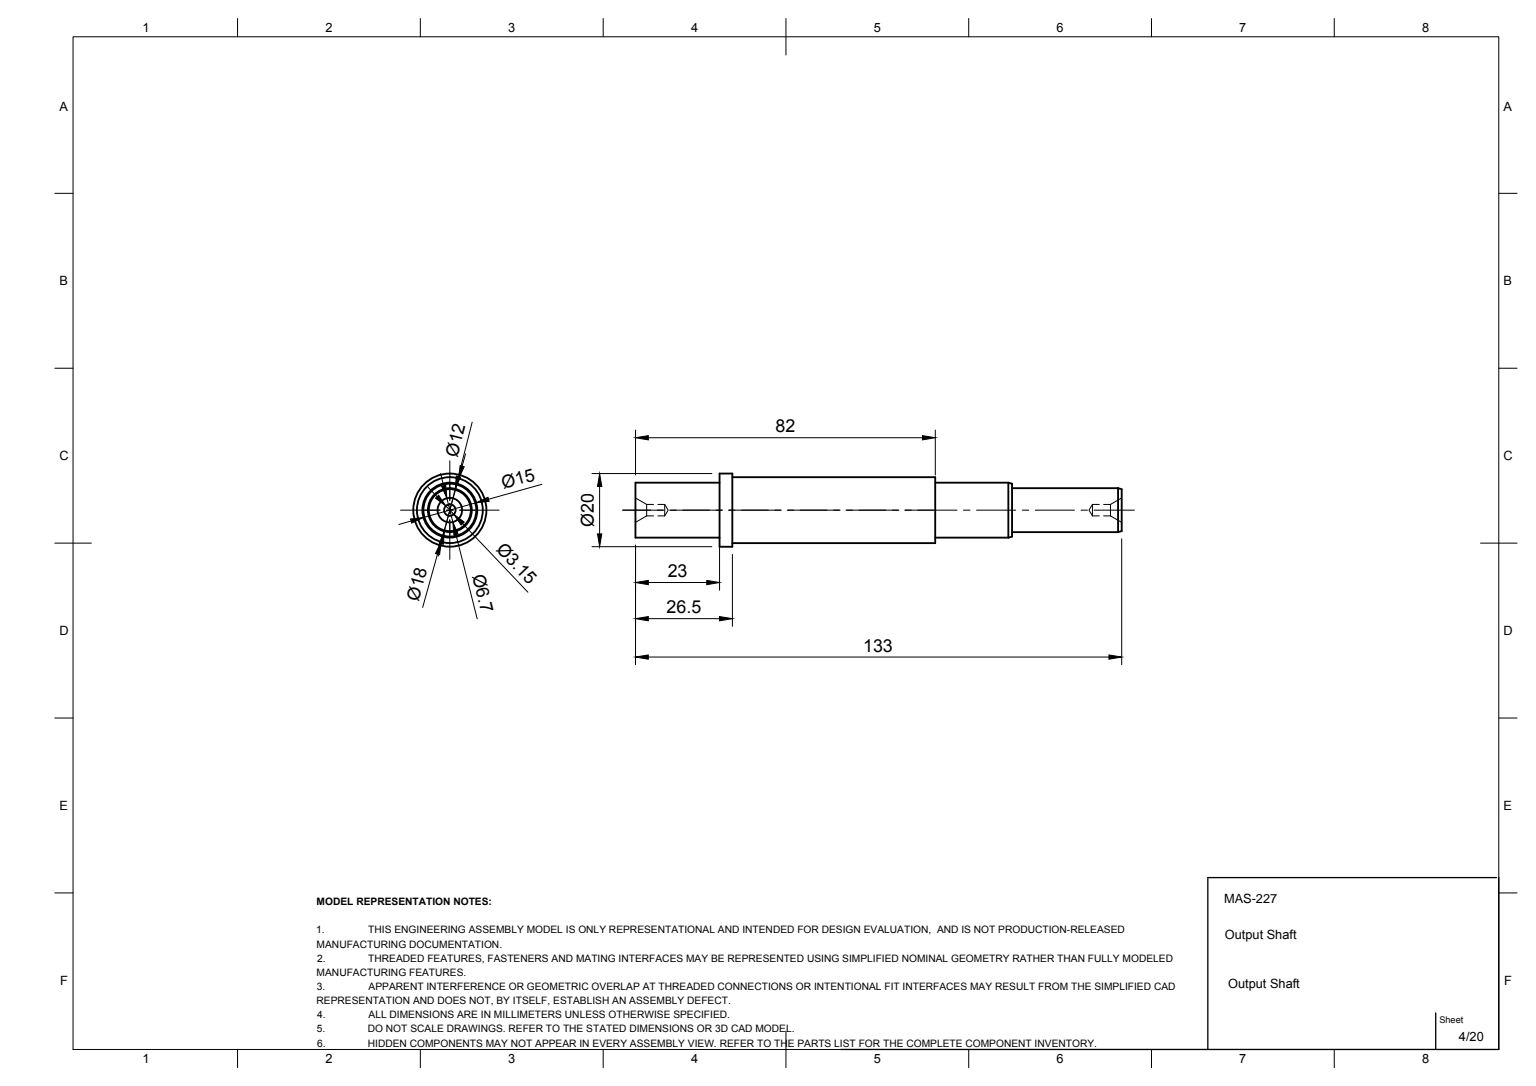
ISO-10303-21;
HEADER;
FILE_DESCRIPTION (('STEP AP214'),
    '1' );
FILE_NAME ( 'Output Shaft.step', '2026-10-06T08:24:41', ( '' ), ( '' ), 'STEP AP214', 'Unspecified', '' );
FILE_SCHEMA (( 'AUTOMOTIVE_DESIGN' ));
ENDSEC;
DATA;
#45=EDGE_CURVE ( 'NONE', #18347, #8484, #23181, .T. ) ;
#57=EDGE_CURVE ( 'NONE', #14897, #14790, #10537, .T. ) ;
#66=DIRECTION ( 'NONE',  ( 0.000000000000000000, 0.000000000000000000, 1.000000000000000000 ) ) ;
#83=DIRECTION ( 'NONE',  ( 0.000000000000000000, 0.000000000000000000, 1.000000000000000000 ) ) ;
#155=CARTESIAN_POINT ( 'NONE',  ( 0.000000000000000000, 0.000000000000000000, 0.9055118110027171596 ) ) ;
#170=CIRCLE ( 'NONE', #27197, 0.2952755905264887182 ) ;
#187=ORIENTED_EDGE ( 'NONE', *, *, #16548, .F. ) ;
#191=ORIENTED_EDGE ( 'NONE', *, *, #12482, .T. ) ;
#231=DIRECTION ( 'NONE',  ( 0.000000000000000000, 0.000000000000000000, 1.000000000000000000 ) ) ;
#281=FACE_OUTER_BOUND ( 'NONE', #3824, .T. ) ;
#333=VERTEX_POINT ( 'NONE', #9774 ) ;
#337=CONICAL_SURFACE ( 'NONE', #25107, 0.06200787401574805319, 1.029744258088332254 ) ;
#346=CARTESIAN_POINT ( 'NONE',  ( 0.06200787401574806013, 0.000000000000000000, 0.7844728274238290666 ) ) ;
#347=ORIENTED_EDGE ( 'NONE', *, *, #11626, .F. ) ;
#395=DIRECTION ( 'NONE',  ( 1.000000000000000000, 0.000000000000000000, 0.000000000000000000 ) ) ;
#427=LINE ( 'NONE', #11141, #5205 ) ;
#455=EDGE_LOOP ( 'NONE', ( #21563, #19160, #191, #7147 ) ) ;
#458=AXIS2_PLACEMENT_3D ( 'NONE', #6185, #12523, #23694 ) ;
#486=DIRECTION ( 'NONE',  ( 1.000000000000000000, 0.000000000000000000, 0.000000000000000000 ) ) ;
#504=LINE ( 'NONE', #11227, #20509 ) ;
#530=CARTESIAN_POINT ( 'NONE',  ( 0.000000000000000000, 0.000000000000000000, -3.110236220451535694 ) ) ;
#576=ORIENTED_EDGE ( 'NONE', *, *, #1922, .T. ) ;
#611=AXIS2_PLACEMENT_3D ( 'NONE', #25131, #20899, #5796 ) ;
#652=CYLINDRICAL_SURFACE ( 'NONE', #15066, 0.2952755905264887182 ) ;
#664=DIRECTION ( 'NONE',  ( 0.000000000000000000, 0.000000000000000000, 1.000000000000000000 ) ) ;
#666=EDGE_CURVE ( 'NONE', #8687, #1454, #4948, .T. ) ;
#667=VECTOR ( 'NONE', #27557, 39.37007874015748143 ) ;
#685=DIRECTION ( 'NONE',  ( 0.000000000000000000, 0.000000000000000000, 1.000000000000000000 ) ) ;
#716=AXIS2_PLACEMENT_3D ( 'NONE', #13335, #23940, #21541 ) ;
#783=VERTEX_POINT ( 'NONE', #2370 ) ;
#786=ORIENTED_EDGE ( 'NONE', *, *, #1340, .T. ) ;
#806=CARTESIAN_POINT ( 'NONE',  ( -0.2952755905264887182, 3.616083068046089993E-17, -4.330708661417323135 ) ) ;
#815=DIRECTION ( 'NONE',  ( 1.000000000000000000, 0.000000000000000000, 0.000000000000000000 ) ) ;
#858=VERTEX_POINT ( 'NONE', #2113 ) ;
#924=DIRECTION ( 'NONE',  ( 1.000000000000000000, 0.000000000000000000, 0.000000000000000000 ) ) ;
#988=DIRECTION ( 'NONE',  ( 1.000000000000000000, 0.000000000000000000, 0.000000000000000000 ) ) ;
#1066=CIRCLE ( 'NONE', #3291, 0.06200787401574806013 ) ;
#1135=CARTESIAN_POINT ( 'NONE',  ( 0.000000000000000000, 0.000000000000000000, -0.1377952755696461029 ) ) ;
#1148=LENGTH_MEASURE_WITH_UNIT ( LENGTH_MEASURE( 0.02539999999999999897 ), #16121 ) ;
#1149=AXIS2_PLACEMENT_3D ( 'NONE', #9958, #18559, #8409 ) ;
#1155=ORIENTED_EDGE ( 'NONE', *, *, #18449, .F. ) ;
#1163=AXIS2_PLACEMENT_3D ( 'NONE', #5767, #10124, #27373 ) ;
#1170=VECTOR ( 'NONE', #19085, 39.37007874015748143 ) ;
#1200=ORIENTED_EDGE ( 'NONE', *, *, #18449, .T. ) ;
#1297=DIRECTION ( 'NONE',  ( 0.000000000000000000, 0.000000000000000000, 1.000000000000000000 ) ) ;
#1299=CARTESIAN_POINT ( 'NONE',  ( 0.3543307086367249448, 0.000000000000000000, -2.322834645648385710 ) ) ;
#1340=EDGE_CURVE ( 'NONE', #2005, #10433, #10148, .T. ) ;
#1368=VECTOR ( 'NONE', #4932, 39.37007874015748143 ) ;
#1388=VERTEX_POINT ( 'NONE', #17057 ) ;
#1454=VERTEX_POINT ( 'NONE', #8971 ) ;
#1460=CARTESIAN_POINT ( 'NONE',  ( -0.2952755905264887182, 3.616083068046089993E-17, -3.110236220451535694 ) ) ;
#1530=ORIENTED_EDGE ( 'NONE', *, *, #9947, .T. ) ;
#1547=DIRECTION ( 'NONE',  ( 0.000000000000000000, 0.000000000000000000, 1.000000000000000000 ) ) ;
#1562=DIRECTION ( 'NONE',  ( 0.000000000000000000, 0.000000000000000000, 1.000000000000000000 ) ) ;
#1604=AXIS2_PLACEMENT_3D ( 'NONE', #9998, #20742, #23148 ) ;
#1728=AXIS2_PLACEMENT_3D ( 'NONE', #26105, #21872, #19190 ) ;
#1815=EDGE_LOOP ( 'NONE', ( #12372, #8684, #25819, #8751 ) ) ;
#1830=ADVANCED_FACE ( 'NONE', ( #7380 ), #27323, .F. ) ;
#1833=LINE ( 'NONE', #12286, #667 ) ;
#1876=EDGE_CURVE ( 'NONE', #10634, #15096, #5263, .T. ) ;
#1890=ORIENTED_EDGE ( 'NONE', *, *, #2911, .F. ) ;
#1922=EDGE_CURVE ( 'NONE', #11128, #20567, #12440, .T. ) ;
#1923=DIRECTION ( 'NONE',  ( 0.000000000000000000, 0.000000000000000000, 1.000000000000000000 ) ) ;
#1948=EDGE_CURVE ( 'NONE', #14897, #8484, #427, .T. ) ;
#2003=ORIENTED_EDGE ( 'NONE', *, *, #14808, .T. ) ;
#2005=VERTEX_POINT ( 'NONE', #5050 ) ;
#2025=DIRECTION ( 'NONE',  ( -0.000000000000000000, 0.000000000000000000, -1.000000000000000000 ) ) ;
#2038=AXIS2_PLACEMENT_3D ( 'NONE', #19503, #66, #8628 ) ;
#2046=VECTOR ( 'NONE', #3128, 39.37007874015748143 ) ;
#2109=ADVANCED_FACE ( 'NONE', ( #3781, #3200 ), #3629, .T. ) ;
#2113=CARTESIAN_POINT ( 'NONE',  ( -0.1318897637674579792, 1.615183770381179830E-17, 0.9055118110027171596 ) ) ;
#2211=CIRCLE ( 'NONE', #10787, 0.2952755905264887182 ) ;
#2257=ORIENTED_EDGE ( 'NONE', *, *, #23536, .F. ) ;
#2258=ADVANCED_FACE ( 'NONE', ( #7995 ), #16600, .F. ) ;
#2260=CARTESIAN_POINT ( 'NONE',  ( 0.2256712916308122319, 0.000000000000000000, -4.330708661396418080 ) ) ;
#2336=ORIENTED_EDGE ( 'NONE', *, *, #12419, .F. ) ;
#2352=ORIENTED_EDGE ( 'NONE', *, *, #6736, .F. ) ;
#2370=CARTESIAN_POINT ( 'NONE',  ( 0.000000000000000000, 0.000000000000000000, 0.5532930914870253236 ) ) ;
#2390=LINE ( 'NONE', #12852, #11209 ) ;
#2402=CARTESIAN_POINT ( 'NONE',  ( -0.2362204724225640262, 2.892866454453686688E-17, -3.149606299191693548 ) ) ;
#2489=ORIENTED_EDGE ( 'NONE', *, *, #20690, .T. ) ;
#2494=ORIENTED_EDGE ( 'NONE', *, *, #666, .T. ) ;
#2545=EDGE_CURVE ( 'NONE', #11128, #16194, #21500, .T. ) ;
#2552=CIRCLE ( 'NONE', #3434, 0.3937007873768824662 ) ;
#2567=VERTEX_POINT ( 'NONE', #17258 ) ;
#2589=CARTESIAN_POINT ( 'NONE',  ( 0.000000000000000000, 0.000000000000000000, -3.110236220451535694 ) ) ;
#2607=CARTESIAN_POINT ( 'NONE',  ( 0.000000000000000000, 0.000000000000000000, -4.015748031496062964 ) ) ;
#2727=DIRECTION ( 'NONE',  ( -1.000000000000000000, 0.000000000000000000, 0.000000000000000000 ) ) ;
#2750=LINE ( 'NONE', #4347, #6018 ) ;
#2779=CIRCLE ( 'NONE', #17251, 0.3543307086367249448 ) ;
#2862=CARTESIAN_POINT ( 'NONE',  ( -0.2952755905264887182, 3.616083068046089993E-17, 2.090519358671640647E-11 ) ) ;
#2911=EDGE_CURVE ( 'NONE', #2567, #858, #13621, .T. ) ;
#2938=DIRECTION ( 'NONE',  ( 0.000000000000000000, 0.000000000000000000, 1.000000000000000000 ) ) ;
#3026=ORIENTED_EDGE ( 'NONE', *, *, #57, .T. ) ;
#3110=MECHANICAL_DESIGN_GEOMETRIC_PRESENTATION_REPRESENTATION('',(#18434),#11231);
#3128=DIRECTION ( 'NONE',  ( 0.4999999999999993894, 6.123233995736758640E-17, -0.8660254037844389297 ) ) ;
#3193=CARTESIAN_POINT ( 'NONE',  ( 0.000000000000000000, 0.000000000000000000, 0.5905511811023621549 ) ) ;
#3200=FACE_BOUND ( 'NONE', #16559, .T. ) ;
#3215=CARTESIAN_POINT ( 'NONE',  ( 0.000000000000000000, 0.000000000000000000, -4.330708661396418080 ) ) ;
#3220=DIRECTION ( 'NONE',  ( 0.000000000000000000, 0.000000000000000000, 1.000000000000000000 ) ) ;
#3240=CIRCLE ( 'NONE', #8236, 0.06200787401574805319 ) ;
#3241=FILL_AREA_STYLE_COLOUR ( '', #9417 ) ;
#3247=VERTEX_POINT ( 'NONE', #22802 ) ;
#3248=ORIENTED_EDGE ( 'NONE', *, *, #16548, .T. ) ;
#3276=ORIENTED_EDGE ( 'NONE', *, *, #6822, .F. ) ;
#3287=DIRECTION ( 'NONE',  ( 1.000000000000000000, 0.000000000000000000, 0.000000000000000000 ) ) ;
#3291=AXIS2_PLACEMENT_3D ( 'NONE', #15788, #13949, #815 ) ;
#3296=ADVANCED_FACE ( 'NONE', ( #22949, #10636 ), #4016, .T. ) ;
#3297=AXIS2_PLACEMENT_3D ( 'NONE', #2589, #11212, #19836 ) ;
#3324=AXIS2_PLACEMENT_3D ( 'NONE', #16852, #21074, #18807 ) ;
#3343=EDGE_CURVE ( 'NONE', #8702, #26390, #17501, .T. ) ;
#3361=ORIENTED_EDGE ( 'NONE', *, *, #23536, .T. ) ;
#3362=DIRECTION ( 'NONE',  ( 0.000000000000000000, 0.000000000000000000, 1.000000000000000000 ) ) ;
#3369=( CONVERSION_BASED_UNIT ( 'INCH', #1148 ) LENGTH_UNIT ( ) NAMED_UNIT ( #6369 ) ) ;
#3381=CIRCLE ( 'NONE', #6159, 0.06200787401574805319 ) ;
#3434=AXIS2_PLACEMENT_3D ( 'NONE', #4019, #23665, #25768 ) ;
#3450=CARTESIAN_POINT ( 'NONE',  ( -0.2256712916308122319, 2.828271352002458705E-17, -4.330708661396418080 ) ) ;
#3451=ORIENTED_EDGE ( 'NONE', *, *, #25299, .T. ) ;
#3487=EDGE_LOOP ( 'NONE', ( #23107, #786 ) ) ;
#3603=ORIENTED_EDGE ( 'NONE', *, *, #1922, .F. ) ;
#3629=PLANE ( 'NONE',  #1604 ) ;
#3651=FACE_OUTER_BOUND ( 'NONE', #18681, .T. ) ;
#3657=DIRECTION ( 'NONE',  ( -0.8571673003991039375, 0.000000000000000000, -0.5150380754143447648 ) ) ;
#3665=DIRECTION ( 'NONE',  ( 0.000000000000000000, 0.000000000000000000, 1.000000000000000000 ) ) ;
#3679=AXIS2_PLACEMENT_3D ( 'NONE', #19825, #10934, #486 ) ;
#3754=DIRECTION ( 'NONE',  ( 0.000000000000000000, 0.000000000000000000, 1.000000000000000000 ) ) ;
#3759=CARTESIAN_POINT ( 'NONE',  ( 0.3543307086367249448, 0.000000000000000000, -2.322834645648386154 ) ) ;
#3764=DIRECTION ( 'NONE',  ( 0.5000000000000009992, 0.000000000000000000, 0.8660254037844380415 ) ) ;
#3781=FACE_OUTER_BOUND ( 'NONE', #9605, .T. ) ;
#3808=CARTESIAN_POINT ( 'NONE',  ( 0.1318897637674579792, 0.000000000000000000, 0.9055118110027171596 ) ) ;
#3824=EDGE_LOOP ( 'NONE', ( #21964, #23743, #16597, #12033 ) ) ;
#3944=ORIENTED_EDGE ( 'NONE', *, *, #4192, .F. ) ;
#4003=CARTESIAN_POINT ( 'NONE',  ( 0.000000000000000000, 0.000000000000000000, -4.330708661396418080 ) ) ;
#4016=PLANE ( 'NONE',  #10735 ) ;
#4019=CARTESIAN_POINT ( 'NONE',  ( 0.000000000000000000, 0.000000000000000000, 2.090519358671640647E-11 ) ) ;
#4103=ORIENTED_EDGE ( 'NONE', *, *, #4417, .F. ) ;
#4119=EDGE_CURVE ( 'NONE', #20567, #11128, #8534, .T. ) ;
#4126=CARTESIAN_POINT ( 'NONE',  ( 0.06200787401574805319, 0.000000000000000000, -4.330708661417323135 ) ) ;
#4144=CIRCLE ( 'NONE', #3679, 0.06200787401574806013 ) ;
#4151=DIRECTION ( 'NONE',  ( -1.000000000000000000, 0.000000000000000000, 0.000000000000000000 ) ) ;
#4160=CYLINDRICAL_SURFACE ( 'NONE', #18408, 0.3543307086367249448 ) ;
#4192=EDGE_CURVE ( 'NONE', #7888, #3247, #4462, .T. ) ;
#4218=DIRECTION ( 'NONE',  ( 0.000000000000000000, 0.000000000000000000, 1.000000000000000000 ) ) ;
#4224=AXIS2_PLACEMENT_3D ( 'NONE', #21526, #25764, #6415 ) ;
#4240=CLOSED_SHELL ( 'NONE', ( #1830, #13050, #19431, #11481, #22826, #19397, #5725, #6414, #10444, #23680, #12611, #27305, #13808, #2258, #26833, #26614, #7641, #9887, #2109, #11451, #4519, #4609, #3296, #5606, #6419, #15626, #14039, #21511, #9703, #11107, #20369, #24480 ) ) ;
#4247=DIRECTION ( 'NONE',  ( -0.000000000000000000, -0.000000000000000000, -1.000000000000000000 ) ) ;
#4257=DIRECTION ( 'NONE',  ( 0.000000000000000000, 0.000000000000000000, 1.000000000000000000 ) ) ;
#4271=ORIENTED_EDGE ( 'NONE', *, *, #15237, .T. ) ;
#4347=CARTESIAN_POINT ( 'NONE',  ( -0.06200787401574805319, 7.593774443531818500E-18, -4.330708661417323135 ) ) ;
#4363=ORIENTED_EDGE ( 'NONE', *, *, #16536, .F. ) ;
#4388=ORIENTED_EDGE ( 'NONE', *, *, #4417, .T. ) ;
#4417=EDGE_CURVE ( 'NONE', #10634, #5423, #18907, .T. ) ;
#4421=DIRECTION ( 'NONE',  ( 1.000000000000000000, 0.000000000000000000, 0.000000000000000000 ) ) ;
#4462=CIRCLE ( 'NONE', #20237, 0.2952755905264887182 ) ;
#4474=VERTEX_POINT ( 'NONE', #8933 ) ;
#4519=ADVANCED_FACE ( 'NONE', ( #8848, #11110 ), #17337, .T. ) ;
#4528=CARTESIAN_POINT ( 'NONE',  ( -0.3937007873768824662, 4.821444090828918336E-17, -4.330708661417323135 ) ) ;
#4554=ORIENTED_EDGE ( 'NONE', *, *, #10365, .T. ) ;
#4606=DIRECTION ( 'NONE',  ( 0.000000000000000000, 0.000000000000000000, 1.000000000000000000 ) ) ;
#4609=ADVANCED_FACE ( 'NONE', ( #24602 ), #24890, .T. ) ;
#4750=DIRECTION ( 'NONE',  ( 0.000000000000000000, 0.000000000000000000, 1.000000000000000000 ) ) ;
#4823=EDGE_CURVE ( 'NONE', #11214, #23414, #20724, .T. ) ;
#4871=VECTOR ( 'NONE', #1562, 39.37007874015748143 ) ;
#4892=DIRECTION ( 'NONE',  ( 0.000000000000000000, 0.000000000000000000, 1.000000000000000000 ) ) ;
#4907=DIRECTION ( 'NONE',  ( 0.000000000000000000, 0.000000000000000000, 1.000000000000000000 ) ) ;
#4932=DIRECTION ( 'NONE',  ( 0.000000000000000000, 0.000000000000000000, 1.000000000000000000 ) ) ;
#4948=LINE ( 'NONE', #27263, #26804 ) ;
#4956=CARTESIAN_POINT ( 'NONE',  ( 0.06200787401574775481, 0.000000000000000000, -4.330708661417323135 ) ) ;
#4996=CARTESIAN_POINT ( 'NONE',  ( 0.000000000000000000, 0.000000000000000000, -4.015748031496062964 ) ) ;
#5050=CARTESIAN_POINT ( 'NONE',  ( -0.2952755905264887182, 3.616083068046089993E-17, -2.322834645648386154 ) ) ;
#5053=ORIENTED_EDGE ( 'NONE', *, *, #16911, .T. ) ;
#5081=CONICAL_SURFACE ( 'NONE', #25851, 0.2952755905264887182, 0.2617993876495733341 ) ;
#5086=CARTESIAN_POINT ( 'NONE',  ( 0.000000000000000000, 0.000000000000000000, 39.92337183164450920 ) ) ;
#5205=VECTOR ( 'NONE', #11552, 39.37007874015748143 ) ;
#5210=DIRECTION ( 'NONE',  ( 1.000000000000000000, 0.000000000000000000, 0.000000000000000000 ) ) ;
#5218=CARTESIAN_POINT ( 'NONE',  ( 0.000000000000000000, 0.000000000000000000, -4.330708661417323135 ) ) ;
#5223=CYLINDRICAL_SURFACE ( 'NONE', #6747, 0.3937007873768824662 ) ;
#5229=CARTESIAN_POINT ( 'NONE',  ( 0.000000000000000000, 0.000000000000000000, 0.000000000000000000 ) ) ;
#5234=DIRECTION ( 'NONE',  ( -1.000000000000000000, 0.000000000000000000, 0.000000000000000000 ) ) ;
#5241=FILL_AREA_STYLE ('',( #3241 ) ) ;
#5263=LINE ( 'NONE', #13881, #2046 ) ;
#5322=AXIS2_PLACEMENT_3D ( 'NONE', #12761, #14484, #20963 ) ;
#5339=VECTOR ( 'NONE', #18152, 39.37007874015748143 ) ;
#5364=CARTESIAN_POINT ( 'NONE',  ( 0.000000000000000000, 0.000000000000000000, -4.330708661396418080 ) ) ;
#5395=DIRECTION ( 'NONE',  ( 1.000000000000000000, 0.000000000000000000, 0.000000000000000000 ) ) ;
#5419=DIRECTION ( 'NONE',  ( 1.000000000000000000, 0.000000000000000000, 0.000000000000000000 ) ) ;
#5423=VERTEX_POINT ( 'NONE', #20161 ) ;
#5546=EDGE_CURVE ( 'NONE', #22287, #8702, #10647, .T. ) ;
#5582=ORIENTED_EDGE ( 'NONE', *, *, #57, .F. ) ;
#5590=CONICAL_SURFACE ( 'NONE', #13249, 0.2952755905264887182, 0.2617993876495733341 ) ;
#5606=ADVANCED_FACE ( 'NONE', ( #27374 ), #4160, .T. ) ;
#5611=DIRECTION ( 'NONE',  ( 0.000000000000000000, 0.000000000000000000, 1.000000000000000000 ) ) ;
#5664=( NAMED_UNIT ( * ) SI_UNIT ( $, .STERADIAN. ) SOLID_ANGLE_UNIT ( ) ) ;
#5697=CARTESIAN_POINT ( 'NONE',  ( -0.2952755905264887182, 3.616083068046089993E-17, 0.9055118110027171596 ) ) ;
#5725=ADVANCED_FACE ( 'NONE', ( #16848 ), #5223, .T. ) ;
#5767=CARTESIAN_POINT ( 'NONE',  ( 0.000000000000000000, 0.000000000000000000, -4.330708661417323135 ) ) ;
#5796=DIRECTION ( 'NONE',  ( 1.000000000000000000, 0.000000000000000000, 0.000000000000000000 ) ) ;
#5862=DIRECTION ( 'NONE',  ( 0.000000000000000000, 0.000000000000000000, 1.000000000000000000 ) ) ;
#5902=LINE ( 'NONE', #23280, #24082 ) ;
#5943=CARTESIAN_POINT ( 'NONE',  ( 0.000000000000000000, 0.000000000000000000, -4.330708661417323135 ) ) ;
#5993=EDGE_LOOP ( 'NONE', ( #15111, #4388, #18053, #21999 ) ) ;
#6018=VECTOR ( 'NONE', #4606, 39.37007874015748143 ) ;
#6059=EDGE_LOOP ( 'NONE', ( #187, #16704, #10312, #27289 ) ) ;
#6113=CARTESIAN_POINT ( 'NONE',  ( -0.3543307086367249448, 4.339299681715786259E-17, -0.1377952755696461029 ) ) ;
#6159=AXIS2_PLACEMENT_3D ( 'NONE', #4996, #22663, #3287 ) ;
#6165=FACE_OUTER_BOUND ( 'NONE', #15846, .T. ) ;
#6185=CARTESIAN_POINT ( 'NONE',  ( 0.000000000000000000, 0.000000000000000000, -4.330708661417323135 ) ) ;
#6265=DIRECTION ( 'NONE',  ( -1.000000000000000000, 0.000000000000000000, 0.000000000000000000 ) ) ;
#6329=DIRECTION ( 'NONE',  ( 0.000000000000000000, 0.000000000000000000, 1.000000000000000000 ) ) ;
#6369=DIMENSIONAL_EXPONENTS ( 1.000000000000000000, 0.000000000000000000, 0.000000000000000000, 0.000000000000000000, 0.000000000000000000, 0.000000000000000000, 0.000000000000000000 ) ;
#6371=LINE ( 'NONE', #4528, #13581 ) ;
#6392=AXIS2_PLACEMENT_3D ( 'NONE', #25997, #19494, #9028 ) ;
#6414=ADVANCED_FACE ( 'NONE', ( #15080 ), #21288, .T. ) ;
#6415=DIRECTION ( 'NONE',  ( 1.000000000000000000, 0.000000000000000000, 0.000000000000000000 ) ) ;
#6419=ADVANCED_FACE ( 'NONE', ( #10676, #12800 ), #27785, .T. ) ;
#6455=DIRECTION ( 'NONE',  ( 1.000000000000000000, 0.000000000000000000, 0.000000000000000000 ) ) ;
#6512=DIRECTION ( 'NONE',  ( -0.2588190448135648802, 3.169619147893076053E-17, 0.9659258263664937116 ) ) ;
#6593=AXIS2_PLACEMENT_3D ( 'NONE', #14220, #18421, #24929 ) ;
#6611=FACE_OUTER_BOUND ( 'NONE', #6786, .T. ) ;
#6655=EDGE_CURVE ( 'NONE', #5423, #1388, #10930, .T. ) ;
#6736=EDGE_CURVE ( 'NONE', #21585, #10762, #19856, .T. ) ;
#6747=AXIS2_PLACEMENT_3D ( 'NONE', #5943, #7635, #27131 ) ;
#6777=EDGE_LOOP ( 'NONE', ( #22873, #2494, #8661 ) ) ;
#6786=EDGE_LOOP ( 'NONE', ( #24548, #7322, #27595, #18756 ) ) ;
#6822=EDGE_CURVE ( 'NONE', #25553, #20290, #18035, .T. ) ;
#6896=PRODUCT_DEFINITION ( 'UNKNOWN', '', #11565, #26900 ) ;
#6902=CIRCLE ( 'NONE', #24475, 0.1318897637674579792 ) ;
#6915=ORIENTED_EDGE ( 'NONE', *, *, #9352, .F. ) ;
#6949=EDGE_CURVE ( 'NONE', #11214, #26700, #14458, .T. ) ;
#7011=DIRECTION ( 'NONE',  ( 0.000000000000000000, 0.000000000000000000, 1.000000000000000000 ) ) ;
#7015=ORIENTED_EDGE ( 'NONE', *, *, #18973, .T. ) ;
#7040=AXIS2_PLACEMENT_3D ( 'NONE', #19213, #4247, #25718 ) ;
#7089=LINE ( 'NONE', #4956, #11983 ) ;
#7094=LENGTH_MEASURE_WITH_UNIT ( LENGTH_MEASURE( 0.02539999999999999897 ), #13574 ) ;
#7097=CARTESIAN_POINT ( 'NONE',  ( 0.2952755905264887182, 0.000000000000000000, -3.110236220451535694 ) ) ;
#7147=ORIENTED_EDGE ( 'NONE', *, *, #1340, .F. ) ;
#7226=ORIENTED_EDGE ( 'NONE', *, *, #20478, .F. ) ;
#7322=ORIENTED_EDGE ( 'NONE', *, *, #2911, .T. ) ;
#7368=CIRCLE ( 'NONE', #4224, 0.2952755905264887182 ) ;
#7380=FACE_OUTER_BOUND ( 'NONE', #25252, .T. ) ;
#7398=EDGE_CURVE ( 'NONE', #8484, #2005, #13795, .T. ) ;
#7454=DIRECTION ( 'NONE',  ( 1.000000000000000000, 0.000000000000000000, 0.000000000000000000 ) ) ;
#7489=CARTESIAN_POINT ( 'NONE',  ( 0.1318897637674583401, 1.615183770381184452E-17, -4.330708661396418080 ) ) ;
#7635=DIRECTION ( 'NONE',  ( 0.000000000000000000, 0.000000000000000000, 1.000000000000000000 ) ) ;
#7641=ADVANCED_FACE ( 'NONE', ( #18723 ), #27360, .F. ) ;
#7688=AXIS2_PLACEMENT_3D ( 'NONE', #12269, #25125, #16378 ) ;
#7691=DIRECTION ( 'NONE',  ( 1.000000000000000000, 0.000000000000000000, 0.000000000000000000 ) ) ;
#7736=DIRECTION ( 'NONE',  ( 1.000000000000000000, 0.000000000000000000, 0.000000000000000000 ) ) ;
#7776=AXIS2_PLACEMENT_3D ( 'NONE', #24950, #5611, #8565 ) ;
#7824=ORIENTED_EDGE ( 'NONE', *, *, #23726, .F. ) ;
#7843=APPLICATION_CONTEXT ( 'automotive_design' ) ;
#7888=VERTEX_POINT ( 'NONE', #2862 ) ;
#7909=ORIENTED_EDGE ( 'NONE', *, *, #23726, .T. ) ;
#7923=DIRECTION ( 'NONE',  ( 1.000000000000000000, 0.000000000000000000, 0.000000000000000000 ) ) ;
#7995=FACE_OUTER_BOUND ( 'NONE', #18966, .T. ) ;
#8073=ORIENTED_EDGE ( 'NONE', *, *, #27737, .T. ) ;
#8104=ORIENTED_EDGE ( 'NONE', *, *, #9352, .T. ) ;
#8147=EDGE_LOOP ( 'NONE', ( #2003, #21102, #8346, #9123 ) ) ;
#8236=AXIS2_PLACEMENT_3D ( 'NONE', #2607, #11230, #924 ) ;
#8270=CONICAL_SURFACE ( 'NONE', #14140, 0.06200787401574806013, 0.5235987755983000369 ) ;
#8284=AXIS2_PLACEMENT_3D ( 'NONE', #1135, #26681, #18041 ) ;
#8309=CARTESIAN_POINT ( 'NONE',  ( -0.2952755905264887182, 3.616083068046089993E-17, -4.330708661417323135 ) ) ;
#8312=ORIENTED_EDGE ( 'NONE', *, *, #3343, .T. ) ;
#8331=ORIENTED_EDGE ( 'NONE', *, *, #23563, .T. ) ;
#8333=FACE_OUTER_BOUND ( 'NONE', #1815, .T. ) ;
#8334=ADVANCED_BREP_SHAPE_REPRESENTATION ( 'Output Shaft', ( #21369, #11588 ), #26943 ) ;
#8346=ORIENTED_EDGE ( 'NONE', *, *, #45, .F. ) ;
#8409=DIRECTION ( 'NONE',  ( 1.000000000000000000, 0.000000000000000000, 0.000000000000000000 ) ) ;
#8484=VERTEX_POINT ( 'NONE', #1460 ) ;
#8534=CIRCLE ( 'NONE', #26537, 0.06200787401574803237 ) ;
#8565=DIRECTION ( 'NONE',  ( 1.000000000000000000, 0.000000000000000000, 0.000000000000000000 ) ) ;
#8581=ORIENTED_EDGE ( 'NONE', *, *, #13011, .T. ) ;
#8628=DIRECTION ( 'NONE',  ( 1.000000000000000000, 0.000000000000000000, 0.000000000000000000 ) ) ;
#8638=CIRCLE ( 'NONE', #6392, 0.3543307086367249448 ) ;
#8651=CARTESIAN_POINT ( 'NONE',  ( -0.2362204724225640262, 2.892866454453686688E-17, -4.291338582656260670 ) ) ;
#8661=ORIENTED_EDGE ( 'NONE', *, *, #13195, .F. ) ;
#8667=DIRECTION ( 'NONE',  ( 1.000000000000000000, 0.000000000000000000, 0.000000000000000000 ) ) ;
#8684=ORIENTED_EDGE ( 'NONE', *, *, #22885, .T. ) ;
#8687=VERTEX_POINT ( 'NONE', #18938 ) ;
#8702=VERTEX_POINT ( 'NONE', #16404 ) ;
#8726=FACE_OUTER_BOUND ( 'NONE', #8147, .T. ) ;
#8751=ORIENTED_EDGE ( 'NONE', *, *, #2545, .F. ) ;
#8758=EDGE_LOOP ( 'NONE', ( #8312, #7015 ) ) ;
#8794=EDGE_CURVE ( 'NONE', #5423, #10634, #15444, .T. ) ;
#8811=AXIS2_PLACEMENT_3D ( 'NONE', #27856, #4257, #18544 ) ;
#8848=FACE_OUTER_BOUND ( 'NONE', #8758, .T. ) ;
#8925=CIRCLE ( 'NONE', #10275, 0.2256712916308122319 ) ;
#8933=CARTESIAN_POINT ( 'NONE',  ( -0.3937007873768824662, 4.821444090828918336E-17, -0.1377952755696461029 ) ) ;
#8971=CARTESIAN_POINT ( 'NONE',  ( -0.06200787401574805319, 7.593774443531818500E-18, -4.015748031496062964 ) ) ;
#8996=EDGE_LOOP ( 'NONE', ( #15266, #11286 ) ) ;
#9002=AXIS2_PLACEMENT_3D ( 'NONE', #22796, #14331, #7691 ) ;
#9028=DIRECTION ( 'NONE',  ( 1.000000000000000000, 0.000000000000000000, 0.000000000000000000 ) ) ;
#9066=VECTOR ( 'NONE', #24497, 39.37007874015748143 ) ;
#9096=DIRECTION ( 'NONE',  ( -0.5000000000000009992, 6.123233995736778362E-17, 0.8660254037844380415 ) ) ;
#9108=PRODUCT_CONTEXT ( 'NONE', #22809, 'mechanical' ) ;
#9123=ORIENTED_EDGE ( 'NONE', *, *, #22606, .F. ) ;
#9146=ORIENTED_EDGE ( 'NONE', *, *, #13195, .T. ) ;
#9182=FACE_OUTER_BOUND ( 'NONE', #21750, .T. ) ;
#9190=SURFACE_STYLE_FILL_AREA ( #5241 ) ;
#9237=CARTESIAN_POINT ( 'NONE',  ( 0.000000000000000000, 0.000000000000000000, -4.330708661396418080 ) ) ;
#9352=EDGE_CURVE ( 'NONE', #13928, #858, #6902, .T. ) ;
#9375=ORIENTED_EDGE ( 'NONE', *, *, #21558, .T. ) ;
#9417=COLOUR_RGB ( '', 0.09019608, 0.27058824, 0.51372549) ;
#9439=FACE_OUTER_BOUND ( 'NONE', #25905, .T. ) ;
#9559=CARTESIAN_POINT ( 'NONE',  ( 0.000000000000000000, 0.000000000000000000, 0.5905511811023621549 ) ) ;
#9602=CARTESIAN_POINT ( 'NONE',  ( 0.2256712916308122319, 0.000000000000000000, -4.330708661396418080 ) ) ;
#9605=EDGE_LOOP ( 'NONE', ( #10989, #10775 ) ) ;
#9637=CARTESIAN_POINT ( 'NONE',  ( 0.000000000000000000, 0.000000000000000000, -4.291338582656260670 ) ) ;
#9703=ADVANCED_FACE ( 'NONE', ( #16580 ), #14339, .T. ) ;
#9707=DIRECTION ( 'NONE',  ( 0.000000000000000000, 0.000000000000000000, 1.000000000000000000 ) ) ;
#9725=ORIENTED_EDGE ( 'NONE', *, *, #666, .F. ) ;
#9741=CYLINDRICAL_SURFACE ( 'NONE', #23621, 0.06200787401574775481 ) ;
#9755=DIRECTION ( 'NONE',  ( -0.000000000000000000, 0.000000000000000000, -1.000000000000000000 ) ) ;
#9774=CARTESIAN_POINT ( 'NONE',  ( -0.3543307086367249448, 4.339299681715786259E-17, -2.322834645648385710 ) ) ;
#9823=EDGE_CURVE ( 'NONE', #3247, #7888, #7368, .T. ) ;
#9853=ORIENTED_EDGE ( 'NONE', *, *, #16536, .T. ) ;
#9887=ADVANCED_FACE ( 'NONE', ( #18068 ), #8270, .F. ) ;
#9947=EDGE_CURVE ( 'NONE', #8687, #24154, #20224, .T. ) ;
#9958=CARTESIAN_POINT ( 'NONE',  ( 0.000000000000000000, 0.000000000000000000, -4.330708661417323135 ) ) ;
#9959=FACE_OUTER_BOUND ( 'NONE', #23656, .T. ) ;
#9990=DIRECTION ( 'NONE',  ( 0.000000000000000000, 0.000000000000000000, 1.000000000000000000 ) ) ;
#9998=CARTESIAN_POINT ( 'NONE',  ( 0.1318897637674579792, 0.000000000000000000, 0.9055118110027171596 ) ) ;
#10007=CONICAL_SURFACE ( 'NONE', #16791, 65.52281417845038902, 1.029744258088330700 ) ;
#10028=ORIENTED_EDGE ( 'NONE', *, *, #3343, .F. ) ;
#10044=CARTESIAN_POINT ( 'NONE',  ( 0.000000000000000000, 0.000000000000000000, -3.149606299191693548 ) ) ;
#10066=ORIENTED_EDGE ( 'NONE', *, *, #17947, .T. ) ;
#10124=DIRECTION ( 'NONE',  ( 0.000000000000000000, 0.000000000000000000, 1.000000000000000000 ) ) ;
#10134=VERTEX_POINT ( 'NONE', #6113 ) ;
#10148=CIRCLE ( 'NONE', #25491, 0.2952755905264887182 ) ;
#10163=DIRECTION ( 'NONE',  ( 1.000000000000000000, 0.000000000000000000, 0.000000000000000000 ) ) ;
#10185=EDGE_LOOP ( 'NONE', ( #12804, #5582 ) ) ;
#10190=EDGE_LOOP ( 'NONE', ( #17326, #18059, #7909, #21996 ) ) ;
#10199=ORIENTED_EDGE ( 'NONE', *, *, #26539, .T. ) ;
#10227=ORIENTED_EDGE ( 'NONE', *, *, #21558, .F. ) ;
#10229=VECTOR ( 'NONE', #22467, 39.37007874015748143 ) ;
#10275=AXIS2_PLACEMENT_3D ( 'NONE', #22450, #18036, #5210 ) ;
#10312=ORIENTED_EDGE ( 'NONE', *, *, #5546, .T. ) ;
#10365=EDGE_CURVE ( 'NONE', #783, #20567, #26963, .T. ) ;
#10433=VERTEX_POINT ( 'NONE', #21721 ) ;
#10437=CARTESIAN_POINT ( 'NONE',  ( 0.06200787401574805319, 0.000000000000000000, -4.015748031496062964 ) ) ;
#10444=ADVANCED_FACE ( 'NONE', ( #6611 ), #26694, .F. ) ;
#10483=DIRECTION ( 'NONE',  ( -0.000000000000000000, -0.000000000000000000, -1.000000000000000000 ) ) ;
#10537=CIRCLE ( 'NONE', #20460, 0.2847264097284254447 ) ;
#10588=FACE_OUTER_BOUND ( 'NONE', #6777, .T. ) ;
#10634=VERTEX_POINT ( 'NONE', #15385 ) ;
#10636=FACE_OUTER_BOUND ( 'NONE', #8996, .T. ) ;
#10647=LINE ( 'NONE', #11827, #14878 ) ;
#10676=FACE_BOUND ( 'NONE', #3487, .T. ) ;
#10678=CARTESIAN_POINT ( 'NONE',  ( 0.000000000000000000, 0.000000000000000000, -3.149606299191693548 ) ) ;
#10733=EDGE_LOOP ( 'NONE', ( #2352, #19796 ) ) ;
#10735=AXIS2_PLACEMENT_3D ( 'NONE', #21104, #2025, #4151 ) ;
#10762=VERTEX_POINT ( 'NONE', #3450 ) ;
#10765=CIRCLE ( 'NONE', #1728, 0.2362204724225640262 ) ;
#10775=ORIENTED_EDGE ( 'NONE', *, *, #18332, .T. ) ;
#10787=AXIS2_PLACEMENT_3D ( 'NONE', #25658, #1923, #27648 ) ;
#10816=DIRECTION ( 'NONE',  ( 1.000000000000000000, 0.000000000000000000, 0.000000000000000000 ) ) ;
#10818=DIRECTION ( 'NONE',  ( 0.000000000000000000, 0.000000000000000000, 1.000000000000000000 ) ) ;
#10930=LINE ( 'NONE', #15972, #13068 ) ;
#10934=DIRECTION ( 'NONE',  ( 0.000000000000000000, 0.000000000000000000, 1.000000000000000000 ) ) ;
#10963=AXIS2_PLACEMENT_3D ( 'NONE', #27535, #4218, #21456 ) ;
#10964=VECTOR ( 'NONE', #24592, 39.37007874015748143 ) ;
#10989=ORIENTED_EDGE ( 'NONE', *, *, #26425, .T. ) ;
#10994=VECTOR ( 'NONE', #20601, 39.37007874015748143 ) ;
#11076=DIRECTION ( 'NONE',  ( 1.000000000000000000, 0.000000000000000000, 0.000000000000000000 ) ) ;
#11107=ADVANCED_FACE ( 'NONE', ( #18089 ), #26287, .T. ) ;
#11110=FACE_BOUND ( 'NONE', #26859, .T. ) ;
#11128=VERTEX_POINT ( 'NONE', #14321 ) ;
#11132=DIRECTION ( 'NONE',  ( 0.000000000000000000, 0.000000000000000000, 1.000000000000000000 ) ) ;
#11141=CARTESIAN_POINT ( 'NONE',  ( -0.2952755905264887182, 3.616083068046089993E-17, -3.110236220451535694 ) ) ;
#11174=CARTESIAN_POINT ( 'NONE',  ( -0.2847264097284254447, 3.551487965556214605E-17, -3.149606299191693548 ) ) ;
#11197=DIRECTION ( 'NONE',  ( 1.000000000000000000, 0.000000000000000000, 0.000000000000000000 ) ) ;
#11209=VECTOR ( 'NONE', #21483, 39.37007874015748143 ) ;
#11212=DIRECTION ( 'NONE',  ( 0.000000000000000000, 0.000000000000000000, 1.000000000000000000 ) ) ;
#11214=VERTEX_POINT ( 'NONE', #8651 ) ;
#11227=CARTESIAN_POINT ( 'NONE',  ( 0.2362204724225640262, 0.000000000000000000, -4.291338582656260670 ) ) ;
#11230=DIRECTION ( 'NONE',  ( 0.000000000000000000, 0.000000000000000000, 1.000000000000000000 ) ) ;
#11231=( GEOMETRIC_REPRESENTATION_CONTEXT ( 3 ) GLOBAL_UNCERTAINTY_ASSIGNED_CONTEXT ( ( #22596 ) ) GLOBAL_UNIT_ASSIGNED_CONTEXT ( ( #15709, #20217, #26705 ) ) REPRESENTATION_CONTEXT ( 'NONE', 'WORKASPACE' ) ) ;
#11240=ORIENTED_EDGE ( 'NONE', *, *, #27737, .F. ) ;
#11286=ORIENTED_EDGE ( 'NONE', *, *, #19746, .F. ) ;
#11451=ADVANCED_FACE ( 'NONE', ( #23586 ), #18893, .T. ) ;
#11453=DIRECTION ( 'NONE',  ( 0.000000000000000000, 0.000000000000000000, 1.000000000000000000 ) ) ;
#11481=ADVANCED_FACE ( 'NONE', ( #8726 ), #5081, .T. ) ;
#11552=DIRECTION ( 'NONE',  ( -0.2588190449580413666, 3.169619149662402932E-17, 0.9659258263277814560 ) ) ;
#11565=PRODUCT_DEFINITION_FORMATION_WITH_SPECIFIED_SOURCE ( 'ANY', '', #24947, .NOT_KNOWN. ) ;
#11588=AXIS2_PLACEMENT_3D ( 'NONE', #5229, #3665, #7923 ) ;
#11626=EDGE_CURVE ( 'NONE', #858, #13928, #15919, .T. ) ;
#11693=CARTESIAN_POINT ( 'NONE',  ( 0.2952755905264887182, 0.000000000000000000, -3.110236220451535694 ) ) ;
#11711=EDGE_LOOP ( 'NONE', ( #12417, #3603, #20959, #12900 ) ) ;
#11755=CARTESIAN_POINT ( 'NONE',  ( 0.000000000000000000, 0.000000000000000000, -4.330708661417323135 ) ) ;
#11763=AXIS2_PLACEMENT_3D ( 'NONE', #14522, #3754, #12375 ) ;
#11795=DIRECTION ( 'NONE',  ( 0.000000000000000000, 0.000000000000000000, 1.000000000000000000 ) ) ;
#11827=CARTESIAN_POINT ( 'NONE',  ( 0.3937007873768824662, 0.000000000000000000, -4.330708661417323135 ) ) ;
#11857=UNCERTAINTY_MEASURE_WITH_UNIT (LENGTH_MEASURE( 1.000000000000000082E-05 ), #3369, 'distance_accuracy_value', 'NONE') ;
#11938=ORIENTED_EDGE ( 'NONE', *, *, #6655, .F. ) ;
#11952=ORIENTED_EDGE ( 'NONE', *, *, #25299, .F. ) ;
#11973=CARTESIAN_POINT ( 'NONE',  ( 0.000000000000000000, 0.000000000000000000, -4.330708661417323135 ) ) ;
#11983=VECTOR ( 'NONE', #11453, 39.37007874015748143 ) ;
#12033=ORIENTED_EDGE ( 'NONE', *, *, #12482, .F. ) ;
#12084=CYLINDRICAL_SURFACE ( 'NONE', #6593, 0.2362204724225640262 ) ;
#12199=CARTESIAN_POINT ( 'NONE',  ( 0.000000000000000000, 0.000000000000000000, -4.330708661417323135 ) ) ;
#12269=CARTESIAN_POINT ( 'NONE',  ( 0.000000000000000000, 0.000000000000000000, -4.291338582656260670 ) ) ;
#12286=CARTESIAN_POINT ( 'NONE',  ( -0.3543307086367249448, 4.339299681715786259E-17, -4.330708661417323135 ) ) ;
#12301=DIRECTION ( 'NONE',  ( -0.000000000000000000, 0.000000000000000000, -1.000000000000000000 ) ) ;
#12306=DIRECTION ( 'NONE',  ( 0.000000000000000000, 0.000000000000000000, 1.000000000000000000 ) ) ;
#12372=ORIENTED_EDGE ( 'NONE', *, *, #4119, .F. ) ;
#12375=DIRECTION ( 'NONE',  ( 1.000000000000000000, 0.000000000000000000, 0.000000000000000000 ) ) ;
#12417=ORIENTED_EDGE ( 'NONE', *, *, #22885, .F. ) ;
#12419=EDGE_CURVE ( 'NONE', #1388, #15096, #15829, .T. ) ;
#12440=CIRCLE ( 'NONE', #26842, 0.06200787401574803237 ) ;
#12482=EDGE_CURVE ( 'NONE', #18347, #10433, #15894, .T. ) ;
#12523=DIRECTION ( 'NONE',  ( 0.000000000000000000, 0.000000000000000000, 1.000000000000000000 ) ) ;
#12611=ADVANCED_FACE ( 'NONE', ( #6165 ), #10007, .F. ) ;
#12612=AXIS2_PLACEMENT_3D ( 'NONE', #12867, #13287, #17388 ) ;
#12637=CARTESIAN_POINT ( 'NONE',  ( 0.000000000000000000, 0.000000000000000000, 39.92337183164450920 ) ) ;
#12647=EDGE_CURVE ( 'NONE', #16194, #2567, #4144, .T. ) ;
#12704=VECTOR ( 'NONE', #6512, 39.37007874015748143 ) ;
#12761=CARTESIAN_POINT ( 'NONE',  ( 0.000000000000000000, 0.000000000000000000, 2.090519358671640647E-11 ) ) ;
#12791=CIRCLE ( 'NONE', #27685, 0.1318897637674583401 ) ;
#12800=FACE_OUTER_BOUND ( 'NONE', #24975, .T. ) ;
#12804=ORIENTED_EDGE ( 'NONE', *, *, #14808, .F. ) ;
#12812=CARTESIAN_POINT ( 'NONE',  ( 0.2952755905264887182, 0.000000000000000000, 2.090530474040783682E-11 ) ) ;
#12826=ORIENTED_EDGE ( 'NONE', *, *, #9823, .T. ) ;
#12848=SHAPE_REPRESENTATION_RELATIONSHIP ( 'NONE' , 'NONE' ,  #13162, #8334 ) ;
#12852=CARTESIAN_POINT ( 'NONE',  ( 2.048885995248197414E-16, 0.000000000000000000, 0.5532930914870255457 ) ) ;
#12867=CARTESIAN_POINT ( 'NONE',  ( 0.000000000000000000, 0.000000000000000000, -4.209669677817527322 ) ) ;
#12900=ORIENTED_EDGE ( 'NONE', *, *, #12647, .T. ) ;
#12906=CONICAL_SURFACE ( 'NONE', #7040, 0.06200787401574805319, 1.029744258088332254 ) ;
#12939=ORIENTED_EDGE ( 'NONE', *, *, #6949, .F. ) ;
#13011=EDGE_CURVE ( 'NONE', #333, #25553, #2779, .T. ) ;
#13050=ADVANCED_FACE ( 'NONE', ( #9439 ), #20853, .T. ) ;
#13068=VECTOR ( 'NONE', #24575, 39.37007874015748143 ) ;
#13096=DIRECTION ( 'NONE',  ( 1.000000000000000000, 0.000000000000000000, 0.000000000000000000 ) ) ;
#13162=SHAPE_REPRESENTATION ( 'Output Shaft', ( #11588 ), #26943 ) ;
#13195=EDGE_CURVE ( 'NONE', #24154, #1454, #3240, .T. ) ;
#13249=AXIS2_PLACEMENT_3D ( 'NONE', #20902, #1547, #27405 ) ;
#13287=DIRECTION ( 'NONE',  ( 0.000000000000000000, 0.000000000000000000, 1.000000000000000000 ) ) ;
#13290=EDGE_LOOP ( 'NONE', ( #9725, #1530, #25757 ) ) ;
#13304=EDGE_CURVE ( 'NONE', #8484, #18347, #170, .T. ) ;
#13335=CARTESIAN_POINT ( 'NONE',  ( 0.000000000000000000, 0.000000000000000000, -0.1377952755696461029 ) ) ;
#13352=CIRCLE ( 'NONE', #716, 0.3937007873768824662 ) ;
#13569=PLANE ( 'NONE',  #21123 ) ;
#13574=( LENGTH_UNIT ( ) NAMED_UNIT ( * ) SI_UNIT ( $, .METRE. ) ) ;
#13581=VECTOR ( 'NONE', #21346, 39.37007874015748143 ) ;
#13621=LINE ( 'NONE', #17973, #25618 ) ;
#13738=DIRECTION ( 'NONE',  ( -1.000000000000000000, 0.000000000000000000, 0.000000000000000000 ) ) ;
#13781=ORIENTED_EDGE ( 'NONE', *, *, #26425, .F. ) ;
#13795=LINE ( 'NONE', #806, #23516 ) ;
#13805=CARTESIAN_POINT ( 'NONE',  ( -0.2362204724225640262, 2.892866454453686688E-17, -4.330708661417323135 ) ) ;
#13808=ADVANCED_FACE ( 'NONE', ( #16109 ), #9741, .F. ) ;
#13864=CARTESIAN_POINT ( 'NONE',  ( 0.06200787401574805319, 7.593774443531818500E-18, -4.015748031496062964 ) ) ;
#13881=CARTESIAN_POINT ( 'NONE',  ( 0.1318897637674583401, 1.615183770381184452E-17, -4.330708661396418080 ) ) ;
#13894=EDGE_LOOP ( 'NONE', ( #24870, #17380 ) ) ;
#13928=VERTEX_POINT ( 'NONE', #3808 ) ;
#13949=DIRECTION ( 'NONE',  ( 0.000000000000000000, 0.000000000000000000, 1.000000000000000000 ) ) ;
#13971=ORIENTED_EDGE ( 'NONE', *, *, #20690, .F. ) ;
#14004=FACE_OUTER_BOUND ( 'NONE', #10733, .T. ) ;
#14039=ADVANCED_FACE ( 'NONE', ( #3651 ), #5590, .T. ) ;
#14140=AXIS2_PLACEMENT_3D ( 'NONE', #20505, #18358, #5395 ) ;
#14144=ORIENTED_EDGE ( 'NONE', *, *, #10365, .F. ) ;
#14154=SURFACE_SIDE_STYLE ('',( #9190 ) ) ;
#14185=DIRECTION ( 'NONE',  ( 0.000000000000000000, 0.000000000000000000, 1.000000000000000000 ) ) ;
#14220=CARTESIAN_POINT ( 'NONE',  ( 0.000000000000000000, 0.000000000000000000, -4.330708661417323135 ) ) ;
#14236=CIRCLE ( 'NONE', #8811, 0.2952755905264887182 ) ;
#14292=ORIENTED_EDGE ( 'NONE', *, *, #1876, .T. ) ;
#14321=CARTESIAN_POINT ( 'NONE',  ( 0.06200787401574803931, 0.000000000000000000, 0.5905511811023621549 ) ) ;
#14331=DIRECTION ( 'NONE',  ( 0.000000000000000000, 0.000000000000000000, 1.000000000000000000 ) ) ;
#14339=CYLINDRICAL_SURFACE ( 'NONE', #24032, 0.2362204724225640262 ) ;
#14390=DIRECTION ( 'NONE',  ( 1.000000000000000000, 0.000000000000000000, 0.000000000000000000 ) ) ;
#14432=EDGE_LOOP ( 'NONE', ( #12826, #8073, #13781, #7226 ) ) ;
#14458=CIRCLE ( 'NONE', #7688, 0.2362204724225640262 ) ;
#14484=DIRECTION ( 'NONE',  ( 0.000000000000000000, 0.000000000000000000, 1.000000000000000000 ) ) ;
#14519=ORIENTED_EDGE ( 'NONE', *, *, #20478, .T. ) ;
#14522=CARTESIAN_POINT ( 'NONE',  ( 0.000000000000000000, 0.000000000000000000, -4.330708661417323135 ) ) ;
#14530=DIRECTION ( 'NONE',  ( 0.000000000000000000, 0.000000000000000000, 1.000000000000000000 ) ) ;
#14543=FACE_OUTER_BOUND ( 'NONE', #455, .T. ) ;
#14549=EDGE_LOOP ( 'NONE', ( #9853, #4271, #2257, #3276 ) ) ;
#14555=CARTESIAN_POINT ( 'NONE',  ( -2.048885995248197414E-16, 2.509161675898543984E-32, 0.5532930914870255457 ) ) ;
#14583=VERTEX_POINT ( 'NONE', #5697 ) ;
#14610=EDGE_LOOP ( 'NONE', ( #11240, #16108, #14519, #17680 ) ) ;
#14711=DIRECTION ( 'NONE',  ( 0.000000000000000000, 0.000000000000000000, 1.000000000000000000 ) ) ;
#14727=CIRCLE ( 'NONE', #2038, 0.3937007873768824662 ) ;
#14790=VERTEX_POINT ( 'NONE', #16705 ) ;
#14808=EDGE_CURVE ( 'NONE', #14790, #14897, #19132, .T. ) ;
#14811=LINE ( 'NONE', #23420, #24746 ) ;
#14878=VECTOR ( 'NONE', #9990, 39.37007874015748143 ) ;
#14897=VERTEX_POINT ( 'NONE', #11174 ) ;
#14945=DIRECTION ( 'NONE',  ( -1.000000000000000000, 0.000000000000000000, 0.000000000000000000 ) ) ;
#15066=AXIS2_PLACEMENT_3D ( 'NONE', #25956, #21854, #19455 ) ;
#15080=FACE_OUTER_BOUND ( 'NONE', #14432, .T. ) ;
#15096=VERTEX_POINT ( 'NONE', #7489 ) ;
#15111=ORIENTED_EDGE ( 'NONE', *, *, #1876, .F. ) ;
#15213=DIRECTION ( 'NONE',  ( 0.2588190448135648802, 0.000000000000000000, 0.9659258263664937116 ) ) ;
#15237=EDGE_CURVE ( 'NONE', #333, #10134, #1833, .T. ) ;
#15266=ORIENTED_EDGE ( 'NONE', *, *, #25931, .F. ) ;
#15366=ORIENTED_EDGE ( 'NONE', *, *, #17665, .T. ) ;
#15385=CARTESIAN_POINT ( 'NONE',  ( 0.06200787401574745644, 0.000000000000000000, -4.209669677817527322 ) ) ;
#15388=ORIENTED_EDGE ( 'NONE', *, *, #1948, .F. ) ;
#15424=LINE ( 'NONE', #25864, #12704 ) ;
#15444=CIRCLE ( 'NONE', #26247, 0.06200787401574745644 ) ;
#15523=AXIS2_PLACEMENT_3D ( 'NONE', #16934, #23849, #13096 ) ;
#15540=LINE ( 'NONE', #11693, #10994 ) ;
#15582=AXIS2_PLACEMENT_3D ( 'NONE', #17727, #7011, #395 ) ;
#15626=ADVANCED_FACE ( 'NONE', ( #14543 ), #22393, .T. ) ;
#15645=ORIENTED_EDGE ( 'NONE', *, *, #6822, .T. ) ;
#15709=( CONVERSION_BASED_UNIT ( 'INCH', #7094 ) LENGTH_UNIT ( ) NAMED_UNIT ( #20779 ) ) ;
#15788=CARTESIAN_POINT ( 'NONE',  ( 0.000000000000000000, 0.000000000000000000, 0.7844728274238290666 ) ) ;
#15829=CIRCLE ( 'NONE', #18067, 0.1318897637674583401 ) ;
#15846=EDGE_LOOP ( 'NONE', ( #13971, #4554, #20002 ) ) ;
#15880=CARTESIAN_POINT ( 'NONE',  ( -0.3937007873768824662, 4.821444090828918336E-17, 2.090519358671640647E-11 ) ) ;
#15894=LINE ( 'NONE', #17856, #9066 ) ;
#15919=CIRCLE ( 'NONE', #20887, 0.1318897637674579792 ) ;
#15972=CARTESIAN_POINT ( 'NONE',  ( -0.1318897637674583401, 0.000000000000000000, -4.330708661396418080 ) ) ;
#16075=DIRECTION ( 'NONE',  ( 1.000000000000000000, 0.000000000000000000, 0.000000000000000000 ) ) ;
#16108=ORIENTED_EDGE ( 'NONE', *, *, #4192, .T. ) ;
#16109=FACE_OUTER_BOUND ( 'NONE', #18924, .T. ) ;
#16121=( LENGTH_UNIT ( ) NAMED_UNIT ( * ) SI_UNIT ( $, .METRE. ) ) ;
#16194=VERTEX_POINT ( 'NONE', #346 ) ;
#16378=DIRECTION ( 'NONE',  ( 1.000000000000000000, 0.000000000000000000, 0.000000000000000000 ) ) ;
#16404=CARTESIAN_POINT ( 'NONE',  ( 0.3937007873768824662, 0.000000000000000000, 2.090519358671640647E-11 ) ) ;
#16456=AXIS2_PLACEMENT_3D ( 'NONE', #10044, #12306, #20931 ) ;
#16512=CYLINDRICAL_SURFACE ( 'NONE', #611, 0.06200787401574805319 ) ;
#16533=FACE_BOUND ( 'NONE', #13894, .T. ) ;
#16536=EDGE_CURVE ( 'NONE', #25553, #333, #8638, .T. ) ;
#16542=EDGE_LOOP ( 'NONE', ( #1890, #27380, #27772, #8104 ) ) ;
#16548=EDGE_CURVE ( 'NONE', #4474, #26390, #6371, .T. ) ;
#16559=EDGE_LOOP ( 'NONE', ( #6915, #347 ) ) ;
#16580=FACE_OUTER_BOUND ( 'NONE', #10190, .T. ) ;
#16597=ORIENTED_EDGE ( 'NONE', *, *, #25911, .F. ) ;
#16600=CYLINDRICAL_SURFACE ( 'NONE', #1149, 0.06200787401574775481 ) ;
#16640=EDGE_LOOP ( 'NONE', ( #19311, #8581, #15645, #25210 ) ) ;
#16704=ORIENTED_EDGE ( 'NONE', *, *, #19746, .T. ) ;
#16705=CARTESIAN_POINT ( 'NONE',  ( 0.2847264097284254447, 0.000000000000000000, -3.149606299191693548 ) ) ;
#16750=FACE_OUTER_BOUND ( 'NONE', #13290, .T. ) ;
#16791=AXIS2_PLACEMENT_3D ( 'NONE', #12637, #21812, #11076 ) ;
#16848=FACE_OUTER_BOUND ( 'NONE', #21935, .T. ) ;
#16852=CARTESIAN_POINT ( 'NONE',  ( 0.000000000000000000, 0.000000000000000000, -3.149606299191693548 ) ) ;
#16911=EDGE_CURVE ( 'NONE', #10134, #20290, #25267, .T. ) ;
#16934=CARTESIAN_POINT ( 'NONE',  ( 0.000000000000000000, 0.000000000000000000, 0.7844728274238290666 ) ) ;
#16971=CARTESIAN_POINT ( 'NONE',  ( 0.2847264097284254447, 0.000000000000000000, -3.149606299191693548 ) ) ;
#17057=CARTESIAN_POINT ( 'NONE',  ( -0.1318897637674583401, 0.000000000000000000, -4.330708661396418080 ) ) ;
#17142=ORIENTED_EDGE ( 'NONE', *, *, #25931, .T. ) ;
#17251=AXIS2_PLACEMENT_3D ( 'NONE', #25237, #14530, #7736 ) ;
#17258=CARTESIAN_POINT ( 'NONE',  ( -0.06200787401574806706, 7.593774443531820041E-18, 0.7844728274238290666 ) ) ;
#17326=ORIENTED_EDGE ( 'NONE', *, *, #4823, .F. ) ;
#17330=CARTESIAN_POINT ( 'NONE',  ( 0.000000000000000000, 0.000000000000000000, -2.322834645648386154 ) ) ;
#17337=PLANE ( 'NONE',  #24706 ) ;
#17380=ORIENTED_EDGE ( 'NONE', *, *, #19297, .T. ) ;
#17388=DIRECTION ( 'NONE',  ( 1.000000000000000000, 0.000000000000000000, 0.000000000000000000 ) ) ;
#17501=CIRCLE ( 'NONE', #5322, 0.3937007873768824662 ) ;
#17665=EDGE_CURVE ( 'NONE', #10762, #21585, #8925, .T. ) ;
#17680=ORIENTED_EDGE ( 'NONE', *, *, #18332, .F. ) ;
#17727=CARTESIAN_POINT ( 'NONE',  ( 0.000000000000000000, 0.000000000000000000, -4.330708661417323135 ) ) ;
#17733=VECTOR ( 'NONE', #11132, 39.37007874015748143 ) ;
#17808=PRESENTATION_STYLE_ASSIGNMENT (( #22755 ) ) ;
#17856=CARTESIAN_POINT ( 'NONE',  ( 0.2952755905264887182, 0.000000000000000000, -4.330708661417323135 ) ) ;
#17947=EDGE_CURVE ( 'NONE', #26700, #11214, #10765, .T. ) ;
#17973=CARTESIAN_POINT ( 'NONE',  ( -0.06200787401574806013, 7.593774443531818500E-18, 0.7844728274238290666 ) ) ;
#18035=LINE ( 'NONE', #24285, #1368 ) ;
#18036=DIRECTION ( 'NONE',  ( 0.000000000000000000, 0.000000000000000000, 1.000000000000000000 ) ) ;
#18041=DIRECTION ( 'NONE',  ( 1.000000000000000000, 0.000000000000000000, 0.000000000000000000 ) ) ;
#18053=ORIENTED_EDGE ( 'NONE', *, *, #6655, .T. ) ;
#18059=ORIENTED_EDGE ( 'NONE', *, *, #6949, .T. ) ;
#18067=AXIS2_PLACEMENT_3D ( 'NONE', #9237, #11795, #20272 ) ;
#18068=FACE_OUTER_BOUND ( 'NONE', #16542, .T. ) ;
#18089=FACE_OUTER_BOUND ( 'NONE', #22667, .T. ) ;
#18152=DIRECTION ( 'NONE',  ( 0.000000000000000000, 0.000000000000000000, 1.000000000000000000 ) ) ;
#18158=DIRECTION ( 'NONE',  ( 1.000000000000000000, 0.000000000000000000, 0.000000000000000000 ) ) ;
#18332=EDGE_CURVE ( 'NONE', #14583, #20609, #2211, .T. ) ;
#18347=VERTEX_POINT ( 'NONE', #7097 ) ;
#18358=DIRECTION ( 'NONE',  ( 0.000000000000000000, 0.000000000000000000, 1.000000000000000000 ) ) ;
#18399=ORIENTED_EDGE ( 'NONE', *, *, #8794, .F. ) ;
#18408=AXIS2_PLACEMENT_3D ( 'NONE', #11973, #25106, #14390 ) ;
#18421=DIRECTION ( 'NONE',  ( 0.000000000000000000, 0.000000000000000000, 1.000000000000000000 ) ) ;
#18434=STYLED_ITEM ( 'NONE', ( #17808 ), #21369 ) ;
#18449=EDGE_CURVE ( 'NONE', #5423, #1454, #14811, .T. ) ;
#18482=DIRECTION ( 'NONE',  ( 1.000000000000000000, 0.000000000000000000, 0.000000000000000000 ) ) ;
#18488=AXIS2_PLACEMENT_3D ( 'NONE', #3215, #2938, #988 ) ;
#18544=DIRECTION ( 'NONE',  ( 1.000000000000000000, 0.000000000000000000, 0.000000000000000000 ) ) ;
#18559=DIRECTION ( 'NONE',  ( 0.000000000000000000, 0.000000000000000000, 1.000000000000000000 ) ) ;
#18633=( NAMED_UNIT ( * ) PLANE_ANGLE_UNIT ( ) SI_UNIT ( $, .RADIAN. ) ) ;
#18636=CARTESIAN_POINT ( 'NONE',  ( 0.2952755905264887182, 0.000000000000000000, 0.9055118110027171596 ) ) ;
#18681=EDGE_LOOP ( 'NONE', ( #15388, #3026, #25604, #25749 ) ) ;
#18723=FACE_OUTER_BOUND ( 'NONE', #11711, .T. ) ;
#18756=ORIENTED_EDGE ( 'NONE', *, *, #23935, .F. ) ;
#18766=AXIS2_PLACEMENT_3D ( 'NONE', #5086, #27273, #10163 ) ;
#18805=ORIENTED_EDGE ( 'NONE', *, *, #26360, .T. ) ;
#18807=DIRECTION ( 'NONE',  ( 1.000000000000000000, 0.000000000000000000, 0.000000000000000000 ) ) ;
#18893=CYLINDRICAL_SURFACE ( 'NONE', #10963, 0.2952755905264887182 ) ;
#18907=CIRCLE ( 'NONE', #12612, 0.06200787401574745644 ) ;
#18924=EDGE_LOOP ( 'NONE', ( #18399, #1200, #18805, #21987 ) ) ;
#18938=CARTESIAN_POINT ( 'NONE',  ( 9.591958661417321355E-18, 0.000000000000000000, -3.978489941880726022 ) ) ;
#18966=EDGE_LOOP ( 'NONE', ( #1155, #4103, #10199, #9146 ) ) ;
#18973=EDGE_CURVE ( 'NONE', #26390, #8702, #2552, .T. ) ;
#19085=DIRECTION ( 'NONE',  ( 0.000000000000000000, 0.000000000000000000, 1.000000000000000000 ) ) ;
#19132=CIRCLE ( 'NONE', #3324, 0.2847264097284254447 ) ;
#19160=ORIENTED_EDGE ( 'NONE', *, *, #13304, .T. ) ;
#19190=DIRECTION ( 'NONE',  ( 1.000000000000000000, 0.000000000000000000, 0.000000000000000000 ) ) ;
#19195=LINE ( 'NONE', #23599, #17733 ) ;
#19213=CARTESIAN_POINT ( 'NONE',  ( 0.000000000000000000, 0.000000000000000000, -4.015748031496062964 ) ) ;
#19265=AXIS2_PLACEMENT_3D ( 'NONE', #10678, #23695, #8667 ) ;
#19297=EDGE_CURVE ( 'NONE', #23414, #27631, #27851, .T. ) ;
#19311=ORIENTED_EDGE ( 'NONE', *, *, #15237, .F. ) ;
#19397=ADVANCED_FACE ( 'NONE', ( #25103 ), #25244, .T. ) ;
#19431=ADVANCED_FACE ( 'NONE', ( #9959 ), #12084, .T. ) ;
#19455=DIRECTION ( 'NONE',  ( 1.000000000000000000, 0.000000000000000000, 0.000000000000000000 ) ) ;
#19486=ORIENTED_EDGE ( 'NONE', *, *, #4823, .T. ) ;
#19494=DIRECTION ( 'NONE',  ( 0.000000000000000000, 0.000000000000000000, 1.000000000000000000 ) ) ;
#19503=CARTESIAN_POINT ( 'NONE',  ( 0.000000000000000000, 0.000000000000000000, -0.1377952755696461029 ) ) ;
#19547=CARTESIAN_POINT ( 'NONE',  ( 0.000000000000000000, 0.000000000000000000, -3.110236220451535694 ) ) ;
#19600=DIRECTION ( 'NONE',  ( 1.000000000000000000, 0.000000000000000000, -0.000000000000000000 ) ) ;
#19614=ORIENTED_EDGE ( 'NONE', *, *, #5546, .F. ) ;
#19746=EDGE_CURVE ( 'NONE', #4474, #22287, #13352, .T. ) ;
#19796=ORIENTED_EDGE ( 'NONE', *, *, #17665, .F. ) ;
#19825=CARTESIAN_POINT ( 'NONE',  ( 0.000000000000000000, 0.000000000000000000, 0.7844728274238290666 ) ) ;
#19836=DIRECTION ( 'NONE',  ( 1.000000000000000000, 0.000000000000000000, 0.000000000000000000 ) ) ;
#19856=CIRCLE ( 'NONE', #18488, 0.2256712916308122319 ) ;
#19858=ORIENTED_EDGE ( 'NONE', *, *, #8794, .T. ) ;
#19965=CARTESIAN_POINT ( 'NONE',  ( 0.3937007873768824662, 0.000000000000000000, -0.1377952755696461029 ) ) ;
#20001=CIRCLE ( 'NONE', #8284, 0.3543307086367249448 ) ;
#20002=ORIENTED_EDGE ( 'NONE', *, *, #4119, .T. ) ;
#20007=DIRECTION ( 'NONE',  ( 1.000000000000000000, 0.000000000000000000, 0.000000000000000000 ) ) ;
#20161=CARTESIAN_POINT ( 'NONE',  ( -0.06200787401574745644, 7.593774443531763034E-18, -4.209669677817527322 ) ) ;
#20204=LINE ( 'NONE', #8309, #10229 ) ;
#20217=( NAMED_UNIT ( * ) PLANE_ANGLE_UNIT ( ) SI_UNIT ( $, .RADIAN. ) ) ;
#20224=LINE ( 'NONE', #13864, #10964 ) ;
#20237=AXIS2_PLACEMENT_3D ( 'NONE', #22281, #4907, #18158 ) ;
#20238=CARTESIAN_POINT ( 'NONE',  ( 0.000000000000000000, 0.000000000000000000, -4.330708661396418080 ) ) ;
#20272=DIRECTION ( 'NONE',  ( 1.000000000000000000, 0.000000000000000000, 0.000000000000000000 ) ) ;
#20290=VERTEX_POINT ( 'NONE', #22473 ) ;
#20369=ADVANCED_FACE ( 'NONE', ( #22053, #14004 ), #13569, .T. ) ;
#20460=AXIS2_PLACEMENT_3D ( 'NONE', #24743, #21707, #26867 ) ;
#20476=DIRECTION ( 'NONE',  ( 1.000000000000000000, 0.000000000000000000, 0.000000000000000000 ) ) ;
#20478=EDGE_CURVE ( 'NONE', #3247, #20609, #22750, .T. ) ;
#20505=CARTESIAN_POINT ( 'NONE',  ( 0.000000000000000000, 0.000000000000000000, 0.7844728274238290666 ) ) ;
#20509=VECTOR ( 'NONE', #15213, 39.37007874015748143 ) ;
#20567=VERTEX_POINT ( 'NONE', #25293 ) ;
#20601=DIRECTION ( 'NONE',  ( 0.2588190449580413666, 0.000000000000000000, 0.9659258263277814560 ) ) ;
#20609=VERTEX_POINT ( 'NONE', #18636 ) ;
#20661=DIRECTION ( 'NONE',  ( -0.000000000000000000, -0.000000000000000000, -1.000000000000000000 ) ) ;
#20690=EDGE_CURVE ( 'NONE', #783, #11128, #2390, .T. ) ;
#20724=LINE ( 'NONE', #13805, #5339 ) ;
#20742=DIRECTION ( 'NONE',  ( 0.000000000000000000, 0.000000000000000000, 1.000000000000000000 ) ) ;
#20779=DIMENSIONAL_EXPONENTS ( 1.000000000000000000, 0.000000000000000000, 0.000000000000000000, 0.000000000000000000, 0.000000000000000000, 0.000000000000000000, 0.000000000000000000 ) ;
#20827=EDGE_LOOP ( 'NONE', ( #22500, #8331 ) ) ;
#20831=SHAPE_DEFINITION_REPRESENTATION ( #26732, #13162 ) ;
#20853=CONICAL_SURFACE ( 'NONE', #7776, 0.2362204724225640262, 0.2617993875000002579 ) ;
#20887=AXIS2_PLACEMENT_3D ( 'NONE', #155, #4892, #20007 ) ;
#20899=DIRECTION ( 'NONE',  ( 0.000000000000000000, 0.000000000000000000, 1.000000000000000000 ) ) ;
#20902=CARTESIAN_POINT ( 'NONE',  ( 0.000000000000000000, 0.000000000000000000, -3.110236220451535694 ) ) ;
#20924=DIRECTION ( 'NONE',  ( -1.000000000000000000, 0.000000000000000000, 0.000000000000000000 ) ) ;
#20931=DIRECTION ( 'NONE',  ( 1.000000000000000000, 0.000000000000000000, 0.000000000000000000 ) ) ;
#20959=ORIENTED_EDGE ( 'NONE', *, *, #2545, .T. ) ;
#20963=DIRECTION ( 'NONE',  ( 1.000000000000000000, 0.000000000000000000, 0.000000000000000000 ) ) ;
#21014=ORIENTED_EDGE ( 'NONE', *, *, #17947, .F. ) ;
#21061=DIRECTION ( 'NONE',  ( 1.000000000000000000, 0.000000000000000000, 0.000000000000000000 ) ) ;
#21074=DIRECTION ( 'NONE',  ( 0.000000000000000000, 0.000000000000000000, 1.000000000000000000 ) ) ;
#21102=ORIENTED_EDGE ( 'NONE', *, *, #1948, .T. ) ;
#21104=CARTESIAN_POINT ( 'NONE',  ( 0.3937007873768824662, 0.000000000000000000, -0.1377952755696460196 ) ) ;
#21123=AXIS2_PLACEMENT_3D ( 'NONE', #9602, #9755, #5234 ) ;
#21209=FACE_OUTER_BOUND ( 'NONE', #10185, .T. ) ;
#21288=CYLINDRICAL_SURFACE ( 'NONE', #458, 0.2952755905264887182 ) ;
#21314=ORIENTED_EDGE ( 'NONE', *, *, #13011, .F. ) ;
#21346=DIRECTION ( 'NONE',  ( 0.000000000000000000, 0.000000000000000000, 1.000000000000000000 ) ) ;
#21369=MANIFOLD_SOLID_BREP ( 'Output Shaft', #4240 ) ;
#21456=DIRECTION ( 'NONE',  ( 1.000000000000000000, 0.000000000000000000, 0.000000000000000000 ) ) ;
#21483=DIRECTION ( 'NONE',  ( 0.8571673003991031603, 0.000000000000000000, 0.5150380754143460971 ) ) ;
#21500=LINE ( 'NONE', #4126, #1170 ) ;
#21511=ADVANCED_FACE ( 'NONE', ( #16533, #21209 ), #27713, .T. ) ;
#21526=CARTESIAN_POINT ( 'NONE',  ( 0.000000000000000000, 0.000000000000000000, 2.090519358671640647E-11 ) ) ;
#21541=DIRECTION ( 'NONE',  ( 1.000000000000000000, 0.000000000000000000, 0.000000000000000000 ) ) ;
#21558=EDGE_CURVE ( 'NONE', #10762, #11214, #15424, .T. ) ;
#21563=ORIENTED_EDGE ( 'NONE', *, *, #7398, .F. ) ;
#21585=VERTEX_POINT ( 'NONE', #2260 ) ;
#21707=DIRECTION ( 'NONE',  ( 0.000000000000000000, 0.000000000000000000, 1.000000000000000000 ) ) ;
#21721=CARTESIAN_POINT ( 'NONE',  ( 0.2952755905264887182, 0.000000000000000000, -2.322834645648386154 ) ) ;
#21726=DIRECTION ( 'NONE',  ( 1.000000000000000000, 0.000000000000000000, 0.000000000000000000 ) ) ;
#21750=EDGE_LOOP ( 'NONE', ( #14144, #2489, #576 ) ) ;
#21812=DIRECTION ( 'NONE',  ( 0.000000000000000000, 0.000000000000000000, 1.000000000000000000 ) ) ;
#21854=DIRECTION ( 'NONE',  ( 0.000000000000000000, 0.000000000000000000, 1.000000000000000000 ) ) ;
#21872=DIRECTION ( 'NONE',  ( 0.000000000000000000, 0.000000000000000000, 1.000000000000000000 ) ) ;
#21935=EDGE_LOOP ( 'NONE', ( #17142, #3248, #10028, #19614 ) ) ;
#21964=ORIENTED_EDGE ( 'NONE', *, *, #45, .T. ) ;
#21987=ORIENTED_EDGE ( 'NONE', *, *, #26539, .F. ) ;
#21996=ORIENTED_EDGE ( 'NONE', *, *, #19297, .F. ) ;
#21999=ORIENTED_EDGE ( 'NONE', *, *, #23563, .F. ) ;
#22053=FACE_BOUND ( 'NONE', #20827, .T. ) ;
#22103=CARTESIAN_POINT ( 'NONE',  ( 0.000000000000000000, 0.000000000000000000, 0.9055118110027171596 ) ) ;
#22133=ORIENTED_EDGE ( 'NONE', *, *, #6736, .T. ) ;
#22281=CARTESIAN_POINT ( 'NONE',  ( 0.000000000000000000, 0.000000000000000000, 2.090519358671640647E-11 ) ) ;
#22287=VERTEX_POINT ( 'NONE', #19965 ) ;
#22393=CYLINDRICAL_SURFACE ( 'NONE', #15582, 0.2952755905264887182 ) ;
#22450=CARTESIAN_POINT ( 'NONE',  ( 0.000000000000000000, 0.000000000000000000, -4.330708661396418080 ) ) ;
#22467=DIRECTION ( 'NONE',  ( 0.000000000000000000, 0.000000000000000000, 1.000000000000000000 ) ) ;
#22473=CARTESIAN_POINT ( 'NONE',  ( 0.3543307086367249448, 0.000000000000000000, -0.1377952755696461029 ) ) ;
#22488=ORIENTED_EDGE ( 'NONE', *, *, #25443, .F. ) ;
#22500=ORIENTED_EDGE ( 'NONE', *, *, #12419, .T. ) ;
#22596=UNCERTAINTY_MEASURE_WITH_UNIT (LENGTH_MEASURE( 1.000000000000000082E-05 ), #15709, 'distance_accuracy_value', 'NONE') ;
#22606=EDGE_CURVE ( 'NONE', #14790, #18347, #15540, .T. ) ;
#22663=DIRECTION ( 'NONE',  ( 0.000000000000000000, 0.000000000000000000, 1.000000000000000000 ) ) ;
#22667=EDGE_LOOP ( 'NONE', ( #10227, #15366, #3451, #12939 ) ) ;
#22718=DIRECTION ( 'NONE',  ( -0.8571673003991031603, 1.049727190767539389E-16, 0.5150380754143460971 ) ) ;
#22750=LINE ( 'NONE', #27275, #4871 ) ;
#22755=SURFACE_STYLE_USAGE ( .BOTH. , #14154 ) ;
#22776=DIRECTION ( 'NONE',  ( 1.000000000000000000, 0.000000000000000000, 0.000000000000000000 ) ) ;
#22796=CARTESIAN_POINT ( 'NONE',  ( 0.000000000000000000, 0.000000000000000000, -0.1377952755696461029 ) ) ;
#22802=CARTESIAN_POINT ( 'NONE',  ( 0.2952755905264887182, 0.000000000000000000, 2.090519358671640647E-11 ) ) ;
#22809=APPLICATION_CONTEXT ( 'automotive_design' ) ;
#22826=ADVANCED_FACE ( 'NONE', ( #281 ), #652, .T. ) ;
#22873=ORIENTED_EDGE ( 'NONE', *, *, #9947, .F. ) ;
#22885=EDGE_CURVE ( 'NONE', #20567, #2567, #2750, .T. ) ;
#22949=FACE_BOUND ( 'NONE', #26387, .T. ) ;
#22951=DIRECTION ( 'NONE',  ( 1.000000000000000000, 0.000000000000000000, 0.000000000000000000 ) ) ;
#23107=ORIENTED_EDGE ( 'NONE', *, *, #25911, .T. ) ;
#23148=DIRECTION ( 'NONE',  ( 1.000000000000000000, 0.000000000000000000, -0.000000000000000000 ) ) ;
#23181=CIRCLE ( 'NONE', #3297, 0.2952755905264887182 ) ;
#23230=CONICAL_SURFACE ( 'NONE', #24095, 0.1318897637674583401, 0.5235987755982981495 ) ;
#23280=CARTESIAN_POINT ( 'NONE',  ( 0.06200787401574806013, 0.000000000000000000, 0.7844728274238290666 ) ) ;
#23323=CONICAL_SURFACE ( 'NONE', #18766, 65.52281417845038902, 1.029744258088330700 ) ;
#23414=VERTEX_POINT ( 'NONE', #2402 ) ;
#23420=CARTESIAN_POINT ( 'NONE',  ( -0.06200787401574775481, 7.593774443531783063E-18, -4.330708661417323135 ) ) ;
#23516=VECTOR ( 'NONE', #664, 39.37007874015748143 ) ;
#23536=EDGE_CURVE ( 'NONE', #20290, #10134, #20001, .T. ) ;
#23563=EDGE_CURVE ( 'NONE', #15096, #1388, #12791, .T. ) ;
#23586=FACE_OUTER_BOUND ( 'NONE', #14610, .T. ) ;
#23599=CARTESIAN_POINT ( 'NONE',  ( 0.2362204724225640262, 0.000000000000000000, -4.330708661417323135 ) ) ;
#23621=AXIS2_PLACEMENT_3D ( 'NONE', #5218, #3362, #18482 ) ;
#23656=EDGE_LOOP ( 'NONE', ( #10066, #19486, #22488, #7824 ) ) ;
#23665=DIRECTION ( 'NONE',  ( 0.000000000000000000, 0.000000000000000000, 1.000000000000000000 ) ) ;
#23680=ADVANCED_FACE ( 'NONE', ( #8333 ), #16512, .F. ) ;
#23694=DIRECTION ( 'NONE',  ( 1.000000000000000000, 0.000000000000000000, 0.000000000000000000 ) ) ;
#23695=DIRECTION ( 'NONE',  ( 0.000000000000000000, 0.000000000000000000, 1.000000000000000000 ) ) ;
#23726=EDGE_CURVE ( 'NONE', #26700, #27631, #19195, .T. ) ;
#23734=CIRCLE ( 'NONE', #24603, 0.2952755905264887182 ) ;
#23743=ORIENTED_EDGE ( 'NONE', *, *, #7398, .T. ) ;
#23839=EDGE_CURVE ( 'NONE', #2567, #16194, #1066, .T. ) ;
#23849=DIRECTION ( 'NONE',  ( 0.000000000000000000, 0.000000000000000000, 1.000000000000000000 ) ) ;
#23917=CARTESIAN_POINT ( 'NONE',  ( 0.000000000000000000, 0.000000000000000000, 0.9055118110027171596 ) ) ;
#23935=EDGE_CURVE ( 'NONE', #16194, #13928, #5902, .T. ) ;
#23940=DIRECTION ( 'NONE',  ( 0.000000000000000000, 0.000000000000000000, 1.000000000000000000 ) ) ;
#24012=VECTOR ( 'NONE', #22718, 39.37007874015748143 ) ;
#24032=AXIS2_PLACEMENT_3D ( 'NONE', #12199, #5862, #22951 ) ;
#24082=VECTOR ( 'NONE', #3764, 39.37007874015748143 ) ;
#24095=AXIS2_PLACEMENT_3D ( 'NONE', #4003, #10483, #6265 ) ;
#24154=VERTEX_POINT ( 'NONE', #10437 ) ;
#24285=CARTESIAN_POINT ( 'NONE',  ( 0.3543307086367249448, 0.000000000000000000, -4.330708661417323135 ) ) ;
#24475=AXIS2_PLACEMENT_3D ( 'NONE', #22103, #14711, #10816 ) ;
#24480=ADVANCED_FACE ( 'NONE', ( #25610 ), #23230, .F. ) ;
#24497=DIRECTION ( 'NONE',  ( 0.000000000000000000, 0.000000000000000000, 1.000000000000000000 ) ) ;
#24548=ORIENTED_EDGE ( 'NONE', *, *, #23839, .F. ) ;
#24575=DIRECTION ( 'NONE',  ( -0.4999999999999993894, 0.000000000000000000, -0.8660254037844389297 ) ) ;
#24592=DIRECTION ( 'NONE',  ( 0.8571673003991039375, 1.049727190767540375E-16, -0.5150380754143447648 ) ) ;
#24602=FACE_OUTER_BOUND ( 'NONE', #6059, .T. ) ;
#24603=AXIS2_PLACEMENT_3D ( 'NONE', #23917, #83, #4421 ) ;
#24706=AXIS2_PLACEMENT_3D ( 'NONE', #12812, #6329, #19600 ) ;
#24743=CARTESIAN_POINT ( 'NONE',  ( 0.000000000000000000, 0.000000000000000000, -3.149606299191693548 ) ) ;
#24746=VECTOR ( 'NONE', #10818, 39.37007874015748143 ) ;
#24870=ORIENTED_EDGE ( 'NONE', *, *, #25443, .T. ) ;
#24890=CYLINDRICAL_SURFACE ( 'NONE', #27500, 0.3937007873768824662 ) ;
#24929=DIRECTION ( 'NONE',  ( 1.000000000000000000, 0.000000000000000000, 0.000000000000000000 ) ) ;
#24947=PRODUCT ( 'Output Shaft', 'Output Shaft', '', ( #9108 ) ) ;
#24950=CARTESIAN_POINT ( 'NONE',  ( 0.000000000000000000, 0.000000000000000000, -4.291338582656260670 ) ) ;
#24975=EDGE_LOOP ( 'NONE', ( #4363, #21314 ) ) ;
#25018=CIRCLE ( 'NONE', #16456, 0.2362204724225640262 ) ;
#25103=FACE_OUTER_BOUND ( 'NONE', #14549, .T. ) ;
#25106=DIRECTION ( 'NONE',  ( 0.000000000000000000, 0.000000000000000000, 1.000000000000000000 ) ) ;
#25107=AXIS2_PLACEMENT_3D ( 'NONE', #27496, #25364, #2727 ) ;
#25125=DIRECTION ( 'NONE',  ( 0.000000000000000000, 0.000000000000000000, 1.000000000000000000 ) ) ;
#25131=CARTESIAN_POINT ( 'NONE',  ( 0.000000000000000000, 0.000000000000000000, -4.330708661417323135 ) ) ;
#25210=ORIENTED_EDGE ( 'NONE', *, *, #16911, .F. ) ;
#25237=CARTESIAN_POINT ( 'NONE',  ( 0.000000000000000000, 0.000000000000000000, -2.322834645648385710 ) ) ;
#25244=CYLINDRICAL_SURFACE ( 'NONE', #1163, 0.3543307086367249448 ) ;
#25252=EDGE_LOOP ( 'NONE', ( #19858, #14292, #2336, #11938 ) ) ;
#25267=CIRCLE ( 'NONE', #9002, 0.3543307086367249448 ) ;
#25293=CARTESIAN_POINT ( 'NONE',  ( -0.06200787401574803931, 7.593774443531816960E-18, 0.5905511811023621549 ) ) ;
#25299=EDGE_CURVE ( 'NONE', #21585, #26700, #504, .T. ) ;
#25364=DIRECTION ( 'NONE',  ( -0.000000000000000000, -0.000000000000000000, -1.000000000000000000 ) ) ;
#25443=EDGE_CURVE ( 'NONE', #27631, #23414, #25018, .T. ) ;
#25491=AXIS2_PLACEMENT_3D ( 'NONE', #17330, #25807, #6455 ) ;
#25553=VERTEX_POINT ( 'NONE', #1299 ) ;
#25604=ORIENTED_EDGE ( 'NONE', *, *, #22606, .T. ) ;
#25610=FACE_OUTER_BOUND ( 'NONE', #5993, .T. ) ;
#25618=VECTOR ( 'NONE', #9096, 39.37007874015748143 ) ;
#25658=CARTESIAN_POINT ( 'NONE',  ( 0.000000000000000000, 0.000000000000000000, 0.9055118110027171596 ) ) ;
#25661=DIRECTION ( 'NONE',  ( -0.000000000000000000, 0.000000000000000000, -1.000000000000000000 ) ) ;
#25677=ORIENTED_EDGE ( 'NONE', *, *, #9823, .F. ) ;
#25718=DIRECTION ( 'NONE',  ( -1.000000000000000000, 0.000000000000000000, 0.000000000000000000 ) ) ;
#25749=ORIENTED_EDGE ( 'NONE', *, *, #13304, .F. ) ;
#25757=ORIENTED_EDGE ( 'NONE', *, *, #26360, .F. ) ;
#25764=DIRECTION ( 'NONE',  ( 0.000000000000000000, 0.000000000000000000, 1.000000000000000000 ) ) ;
#25768=DIRECTION ( 'NONE',  ( 1.000000000000000000, 0.000000000000000000, 0.000000000000000000 ) ) ;
#25807=DIRECTION ( 'NONE',  ( 0.000000000000000000, 0.000000000000000000, 1.000000000000000000 ) ) ;
#25819=ORIENTED_EDGE ( 'NONE', *, *, #23839, .T. ) ;
#25837=AXIS2_PLACEMENT_3D ( 'NONE', #9637, #14185, #5419 ) ;
#25851=AXIS2_PLACEMENT_3D ( 'NONE', #530, #4750, #21726 ) ;
#25864=CARTESIAN_POINT ( 'NONE',  ( -0.2362204724225640262, 2.892866454453686688E-17, -4.291338582656260670 ) ) ;
#25905=EDGE_LOOP ( 'NONE', ( #22133, #9375, #21014, #11952 ) ) ;
#25911=EDGE_CURVE ( 'NONE', #10433, #2005, #14236, .T. ) ;
#25931=EDGE_CURVE ( 'NONE', #22287, #4474, #14727, .T. ) ;
#25956=CARTESIAN_POINT ( 'NONE',  ( 0.000000000000000000, 0.000000000000000000, -4.330708661417323135 ) ) ;
#25977=AXIS2_PLACEMENT_3D ( 'NONE', #20238, #20661, #13738 ) ;
#25997=CARTESIAN_POINT ( 'NONE',  ( 0.000000000000000000, 0.000000000000000000, -2.322834645648385710 ) ) ;
#25999=CARTESIAN_POINT ( 'NONE',  ( 0.2362204724225640262, 0.000000000000000000, -3.149606299191693548 ) ) ;
#26105=CARTESIAN_POINT ( 'NONE',  ( 0.000000000000000000, 0.000000000000000000, -4.291338582656260670 ) ) ;
#26247=AXIS2_PLACEMENT_3D ( 'NONE', #27150, #1297, #21061 ) ;
#26287=CONICAL_SURFACE ( 'NONE', #25837, 0.2362204724225640262, 0.2617993875000002579 ) ;
#26360=EDGE_CURVE ( 'NONE', #1454, #24154, #3381, .T. ) ;
#26387=EDGE_LOOP ( 'NONE', ( #3361, #5053 ) ) ;
#26390=VERTEX_POINT ( 'NONE', #15880 ) ;
#26425=EDGE_CURVE ( 'NONE', #20609, #14583, #23734, .T. ) ;
#26537=AXIS2_PLACEMENT_3D ( 'NONE', #3193, #9707, #16075 ) ;
#26539=EDGE_CURVE ( 'NONE', #10634, #24154, #7089, .T. ) ;
#26573=AXIS2_PLACEMENT_3D ( 'NONE', #3759, #25661, #14945 ) ;
#26614=ADVANCED_FACE ( 'NONE', ( #9182 ), #23323, .F. ) ;
#26681=DIRECTION ( 'NONE',  ( 0.000000000000000000, 0.000000000000000000, 1.000000000000000000 ) ) ;
#26694=CONICAL_SURFACE ( 'NONE', #15523, 0.06200787401574806013, 0.5235987755983000369 ) ;
#26700=VERTEX_POINT ( 'NONE', #27141 ) ;
#26705=( NAMED_UNIT ( * ) SI_UNIT ( $, .STERADIAN. ) SOLID_ANGLE_UNIT ( ) ) ;
#26722=DIRECTION ( 'NONE',  ( 0.000000000000000000, 0.000000000000000000, 1.000000000000000000 ) ) ;
#26732=PRODUCT_DEFINITION_SHAPE ( 'NONE', 'NONE',  #6896 ) ;
#26804=VECTOR ( 'NONE', #3657, 39.37007874015748143 ) ;
#26833=ADVANCED_FACE ( 'NONE', ( #10588 ), #12906, .F. ) ;
#26842=AXIS2_PLACEMENT_3D ( 'NONE', #9559, #685, #7454 ) ;
#26859=EDGE_LOOP ( 'NONE', ( #25677, #3944 ) ) ;
#26867=DIRECTION ( 'NONE',  ( 1.000000000000000000, 0.000000000000000000, 0.000000000000000000 ) ) ;
#26900=PRODUCT_DEFINITION_CONTEXT ( 'detailed design', #7843, 'design' ) ;
#26943=( GEOMETRIC_REPRESENTATION_CONTEXT ( 3 ) GLOBAL_UNCERTAINTY_ASSIGNED_CONTEXT ( ( #11857 ) ) GLOBAL_UNIT_ASSIGNED_CONTEXT ( ( #3369, #18633, #5664 ) ) REPRESENTATION_CONTEXT ( 'NONE', 'WORKASPACE' ) ) ;
#26963=LINE ( 'NONE', #14555, #24012 ) ;
#27131=DIRECTION ( 'NONE',  ( 1.000000000000000000, 0.000000000000000000, 0.000000000000000000 ) ) ;
#27141=CARTESIAN_POINT ( 'NONE',  ( 0.2362204724225640262, 0.000000000000000000, -4.291338582656260670 ) ) ;
#27150=CARTESIAN_POINT ( 'NONE',  ( 0.000000000000000000, 0.000000000000000000, -4.209669677817527322 ) ) ;
#27152=AXIS2_PLACEMENT_3D ( 'NONE', #16971, #12301, #20924 ) ;
#27197=AXIS2_PLACEMENT_3D ( 'NONE', #19547, #231, #11197 ) ;
#27263=CARTESIAN_POINT ( 'NONE',  ( -0.06200787401574805319, 0.000000000000000000, -4.015748031496062964 ) ) ;
#27273=DIRECTION ( 'NONE',  ( 0.000000000000000000, 0.000000000000000000, 1.000000000000000000 ) ) ;
#27275=CARTESIAN_POINT ( 'NONE',  ( 0.2952755905264887182, 0.000000000000000000, -4.330708661417323135 ) ) ;
#27289=ORIENTED_EDGE ( 'NONE', *, *, #18973, .F. ) ;
#27305=ADVANCED_FACE ( 'NONE', ( #16750 ), #337, .F. ) ;
#27323=CONICAL_SURFACE ( 'NONE', #25977, 0.1318897637674583401, 0.5235987755982981495 ) ;
#27360=CYLINDRICAL_SURFACE ( 'NONE', #11763, 0.06200787401574805319 ) ;
#27373=DIRECTION ( 'NONE',  ( 1.000000000000000000, 0.000000000000000000, 0.000000000000000000 ) ) ;
#27374=FACE_OUTER_BOUND ( 'NONE', #16640, .T. ) ;
#27380=ORIENTED_EDGE ( 'NONE', *, *, #12647, .F. ) ;
#27405=DIRECTION ( 'NONE',  ( 1.000000000000000000, 0.000000000000000000, 0.000000000000000000 ) ) ;
#27496=CARTESIAN_POINT ( 'NONE',  ( 0.000000000000000000, 0.000000000000000000, -4.015748031496062964 ) ) ;
#27500=AXIS2_PLACEMENT_3D ( 'NONE', #11755, #26722, #22776 ) ;
#27535=CARTESIAN_POINT ( 'NONE',  ( 0.000000000000000000, 0.000000000000000000, -4.330708661417323135 ) ) ;
#27557=DIRECTION ( 'NONE',  ( 0.000000000000000000, 0.000000000000000000, 1.000000000000000000 ) ) ;
#27595=ORIENTED_EDGE ( 'NONE', *, *, #11626, .T. ) ;
#27631=VERTEX_POINT ( 'NONE', #25999 ) ;
#27648=DIRECTION ( 'NONE',  ( 1.000000000000000000, 0.000000000000000000, 0.000000000000000000 ) ) ;
#27685=AXIS2_PLACEMENT_3D ( 'NONE', #5364, #3220, #20476 ) ;
#27713=PLANE ( 'NONE',  #27152 ) ;
#27737=EDGE_CURVE ( 'NONE', #7888, #14583, #20204, .T. ) ;
#27772=ORIENTED_EDGE ( 'NONE', *, *, #23935, .T. ) ;
#27785=PLANE ( 'NONE',  #26573 ) ;
#27851=CIRCLE ( 'NONE', #19265, 0.2362204724225640262 ) ;
#27856=CARTESIAN_POINT ( 'NONE',  ( 0.000000000000000000, 0.000000000000000000, -2.322834645648386154 ) ) ;
ENDSEC;
END-ISO-10303-21;
